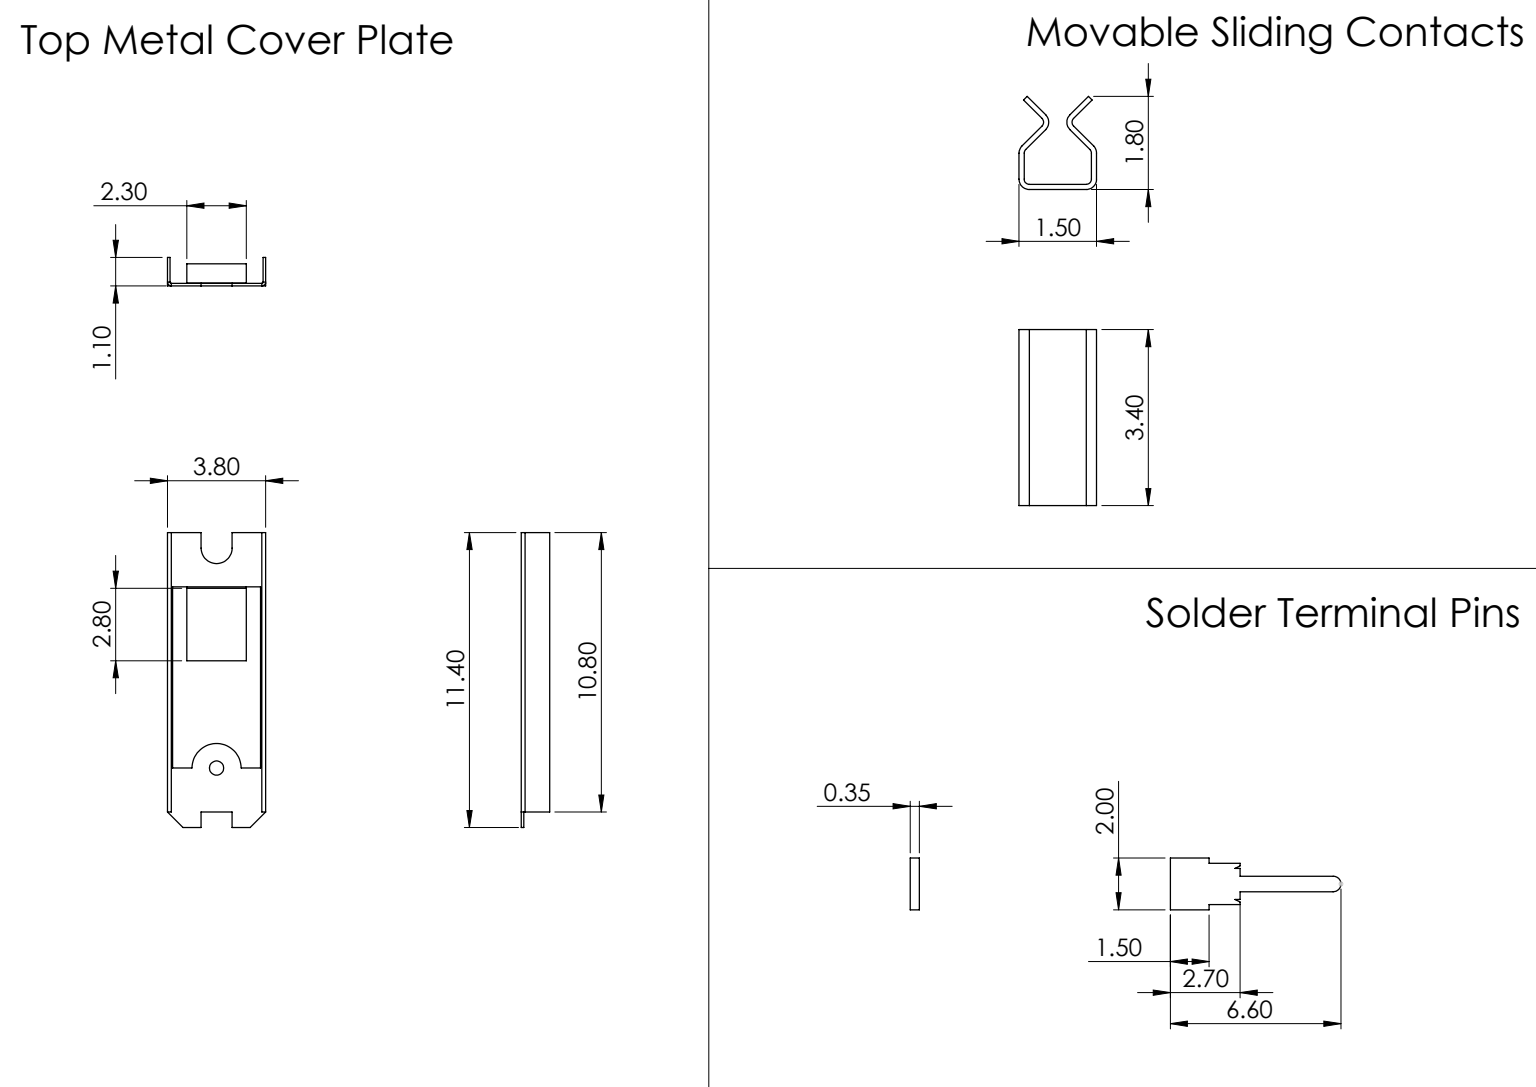
ISO-10303-21;
HEADER;
FILE_DESCRIPTION (('STEP AP214'),
    '1' );
FILE_NAME ('Movable Sliding Contacts.step',
    '2026-10-09T19:32:29',
    ( '' ),
    ( '' ),
    'SwSTEP 2.0',
    'SolidWorks 2026',
    '' );
FILE_SCHEMA (( 'AUTOMOTIVE_DESIGN' ));
ENDSEC;

DATA;
#11=DIRECTION ( 'NONE',  ( 1.306144734853129823E-16, -1.000000000000000000, -1.306144734853129823E-16 ) ) ;
#19=ORIENTED_EDGE ( 'NONE', *, *, #12813, .F. ) ;
#25=CARTESIAN_POINT ( 'NONE',  ( 0.3750000000000000000, 6.450000000000000178, 2.100000000000000089 ) ) ;
#54=CARTESIAN_POINT ( 'NONE',  ( 0.5500000000000000444, 6.450000000000000178, 3.399999999999999911 ) ) ;
#63=FACE_OUTER_BOUND ( 'NONE', #13945, .T. ) ;
#72=ORIENTED_EDGE ( 'NONE', *, *, #16562, .F. ) ;
#74=CARTESIAN_POINT ( 'NONE',  ( 0.5500000000000000444, 6.450000000000000178, 3.200000000000000178 ) ) ;
#100=DIRECTION ( 'NONE',  ( 1.306144734853129823E-16, -1.000000000000000000, -1.306144734853129823E-16 ) ) ;
#143=DIRECTION ( 'NONE',  ( 0.000000000000000000, -1.000000000000000000, -1.306144734853125878E-16 ) ) ;
#164=EDGE_LOOP ( 'NONE', ( #16318, #961, #5589, #9306 ) ) ;
#166=DIRECTION ( 'NONE',  ( 1.000000000000000000, 1.306144734853129823E-16, 0.000000000000000000 ) ) ;
#181=ORIENTED_EDGE ( 'NONE', *, *, #15801, .T. ) ;
#184=AXIS2_PLACEMENT_3D ( 'NONE', #11103, #16750, #840 ) ;
#200=FACE_OUTER_BOUND ( 'NONE', #10573, .T. ) ;
#206=DIRECTION ( 'NONE',  ( 1.142876642996489981E-16, -1.000000000000000000, -6.530723674265629391E-17 ) ) ;
#218=AXIS2_PLACEMENT_3D ( 'NONE', #8248, #6936, #4241 ) ;
#246=VECTOR ( 'NONE', #2226, 1000.000000000000000 ) ;
#258=ORIENTED_EDGE ( 'NONE', *, *, #12874, .T. ) ;
#268=VERTEX_POINT ( 'NONE', #877 ) ;
#269=LINE ( 'NONE', #7559, #15424 ) ;
#314=ORIENTED_EDGE ( 'NONE', *, *, #15602, .T. ) ;
#322=EDGE_CURVE ( 'NONE', #6911, #16493, #5032, .T. ) ;
#340=EDGE_CURVE ( 'NONE', #11433, #9105, #9389, .T. ) ;
#345=ORIENTED_EDGE ( 'NONE', *, *, #10185, .F. ) ;
#353=ORIENTED_EDGE ( 'NONE', *, *, #5292, .T. ) ;
#382=DIRECTION ( 'NONE',  ( 1.000000000000000000, 0.000000000000000000, 0.000000000000000000 ) ) ;
#433=CARTESIAN_POINT ( 'NONE',  ( 0.6207106781186549904, 3.050000000000000266, 2.628553390593269423 ) ) ;
#472=ADVANCED_FACE ( 'NONE', ( #11019 ), #9341, .T. ) ;
#507=CARTESIAN_POINT ( 'NONE',  ( -0.3750000000000000000, 3.050000000000000266, 2.100000000000000089 ) ) ;
#552=( GEOMETRIC_REPRESENTATION_CONTEXT ( 3 ) GLOBAL_UNCERTAINTY_ASSIGNED_CONTEXT ( ( #2517 ) ) GLOBAL_UNIT_ASSIGNED_CONTEXT ( ( #4504, #3040, #6174 ) ) REPRESENTATION_CONTEXT ( 'NONE', 'WORKASPACE' ) );
#554=DIRECTION ( 'NONE',  ( 1.306144734853129823E-16, -1.000000000000000000, -6.530723674265629391E-17 ) ) ;
#561=ADVANCED_FACE ( 'NONE', ( #4065 ), #6855, .F. ) ;
#606=CIRCLE ( 'NONE', #11850, 0.1999999999999999833 ) ;
#658=CARTESIAN_POINT ( 'NONE',  ( 0.6628679656440349399, 3.050000000000000266, 1.670710678118660031 ) ) ;
#668=DIRECTION ( 'NONE',  ( 0.7071067811865466846, 0.000000000000000000, -0.7071067811865483499 ) ) ;
#671=ORIENTED_EDGE ( 'NONE', *, *, #7463, .F. ) ;
#683=DIRECTION ( 'NONE',  ( 1.224646799147350002E-16, -1.000000000000000000, -6.123233995736769734E-17 ) ) ;
#686=ADVANCED_BREP_SHAPE_REPRESENTATION ( '', ( #7724, #17681 ), #552 ) ;
#696=PLANE ( 'NONE',  #836 ) ;
#706=ORIENTED_EDGE ( 'NONE', *, *, #14653, .F. ) ;
#724=ORIENTED_EDGE ( 'NONE', *, *, #11762, .T. ) ;
#741=EDGE_CURVE ( 'NONE', #9183, #17652, #3050, .T. ) ;
#758=EDGE_CURVE ( 'NONE', #16493, #14177, #16933, .T. ) ;
#771=VECTOR ( 'NONE', #10141, 1000.000000000000000 ) ;
#836=AXIS2_PLACEMENT_3D ( 'NONE', #6620, #6332, #10894 ) ;
#840=DIRECTION ( 'NONE',  ( 0.7071067811865594521, 0.000000000000000000, 0.7071067811865355823 ) ) ;
#845=ORIENTED_EDGE ( 'NONE', *, *, #5292, .F. ) ;
#877=CARTESIAN_POINT ( 'NONE',  ( 0.3042893218813449985, 3.050000000000000266, 2.170710678118660031 ) ) ;
#886=DIRECTION ( 'NONE',  ( -1.000000000000000000, 0.000000000000000000, 0.000000000000000000 ) ) ;
#931=FACE_OUTER_BOUND ( 'NONE', #3401, .T. ) ;
#949=CARTESIAN_POINT ( 'NONE',  ( -0.3042893218813459977, 6.450000000000000178, 2.029289321881350361 ) ) ;
#961=ORIENTED_EDGE ( 'NONE', *, *, #14653, .T. ) ;
#968=AXIS2_PLACEMENT_3D ( 'NONE', #5506, #11151, #6990 ) ;
#1018=ORIENTED_EDGE ( 'NONE', *, *, #16662, .T. ) ;
#1020=CARTESIAN_POINT ( 'NONE',  ( 0.6500000000000000222, 3.050000000000000266, 2.699264068711930253 ) ) ;
#1038=UNCERTAINTY_MEASURE_WITH_UNIT (LENGTH_MEASURE( 1.000000000000000082E-05 ), #15942, 'distance_accuracy_value', 'NONE');
#1043=CARTESIAN_POINT ( 'NONE',  ( -0.2335786437626909962, 6.450000000000000178, 2.241421356237310203 ) ) ;
#1070=DIRECTION ( 'NONE',  ( -1.224646799147351975E-16, 1.000000000000000000, 6.123233995736759873E-17 ) ) ;
#1079=LINE ( 'NONE', #17619, #15708 ) ;
#1081=DIRECTION ( 'NONE',  ( -1.224646799147350002E-16, 1.000000000000000000, 6.123233995736759873E-17 ) ) ;
#1100=VECTOR ( 'NONE', #13955, 1000.000000000000000 ) ;
#1118=CIRCLE ( 'NONE', #2598, 0.1000000000000000472 ) ;
#1147=ORIENTED_EDGE ( 'NONE', *, *, #10999, .T. ) ;
#1174=DIRECTION ( 'NONE',  ( -0.7071067811865475727, -4.040679121612663150E-17, -0.7071067811865475727 ) ) ;
#1182=DIRECTION ( 'NONE',  ( 1.000000000000000000, 0.000000000000000000, 0.000000000000000000 ) ) ;
#1198=CARTESIAN_POINT ( 'NONE',  ( -0.2335786437626909962, 6.450000000000000178, 2.241421356237310203 ) ) ;
#1199=ORIENTED_EDGE ( 'NONE', *, *, #2728, .T. ) ;
#1200=VECTOR ( 'NONE', #13384, 1000.000000000000000 ) ;
#1213=ADVANCED_FACE ( 'NONE', ( #2544 ), #12549, .T. ) ;
#1248=ORIENTED_EDGE ( 'NONE', *, *, #10846, .F. ) ;
#1251=DIRECTION ( 'NONE',  ( 0.7071067811865470176, -5.772398745161022854E-18, 0.7071067811865480168 ) ) ;
#1258=EDGE_CURVE ( 'NONE', #16824, #6139, #11523, .T. ) ;
#1283=ORIENTED_EDGE ( 'NONE', *, *, #4749, .F. ) ;
#1293=DIRECTION ( 'NONE',  ( -0.7071067811865475727, -4.617918996128746176E-17, -0.7071067811865475727 ) ) ;
#1324=ORIENTED_EDGE ( 'NONE', *, *, #3238, .F. ) ;
#1355=CARTESIAN_POINT ( 'NONE',  ( 0.5500000000000000444, 6.450000000000000178, 3.200000000000000178 ) ) ;
#1378=CARTESIAN_POINT ( 'NONE',  ( 0.6207106781186539912, 6.450000000000000178, 2.628553390593269423 ) ) ;
#1387=ORIENTED_EDGE ( 'NONE', *, *, #18174, .F. ) ;
#1400=AXIS2_PLACEMENT_3D ( 'NONE', #14762, #10784, #13285 ) ;
#1402=CIRCLE ( 'NONE', #3436, 0.2000000000000000389 ) ;
#1451=CARTESIAN_POINT ( 'NONE',  ( 0.6500000000000000222, 6.450000000000000178, 3.200000000000000178 ) ) ;
#1465=FACE_OUTER_BOUND ( 'NONE', #13748, .T. ) ;
#1483=VECTOR ( 'NONE', #3233, 1000.000000000000000 ) ;
#1498=ORIENTED_EDGE ( 'NONE', *, *, #12674, .T. ) ;
#1525=VECTOR ( 'NONE', #14731, 1000.000000000000000 ) ;
#1571=LINE ( 'NONE', #3365, #11024 ) ;
#1587=CARTESIAN_POINT ( 'NONE',  ( 0.5500000000000000444, 3.050000000000000266, 2.699264068711930253 ) ) ;
#1596=DIRECTION ( 'NONE',  ( -1.224646799147350002E-16, 1.000000000000000000, 6.123233995736759873E-17 ) ) ;
#1598=EDGE_CURVE ( 'NONE', #17652, #5170, #13115, .T. ) ;
#1676=DIRECTION ( 'NONE',  ( -1.224646799147350002E-16, 1.000000000000000000, 6.123233995736769734E-17 ) ) ;
#1749=CIRCLE ( 'NONE', #15946, 0.1000000000000000472 ) ;
#1753=DIRECTION ( 'NONE',  ( 1.306144734853129823E-16, -1.000000000000000000, -1.306144734853129823E-16 ) ) ;
#1766=ORIENTED_EDGE ( 'NONE', *, *, #11413, .T. ) ;
#1810=DIRECTION ( 'NONE',  ( 1.306144734853129823E-16, -1.000000000000000000, -1.306144734853129823E-16 ) ) ;
#1814=CARTESIAN_POINT ( 'NONE',  ( -0.5921572875253819923, 6.450000000000000178, 1.600000000000000089 ) ) ;
#1822=EDGE_CURVE ( 'NONE', #12759, #5909, #10605, .T. ) ;
#1842=DIRECTION ( 'NONE',  ( -0.7071067811865470176, 0.000000000000000000, -0.7071067811865480168 ) ) ;
#1881=EDGE_LOOP ( 'NONE', ( #8557, #7086, #17262, #671 ) ) ;
#1892=ORIENTED_EDGE ( 'NONE', *, *, #340, .T. ) ;
#1896=EDGE_CURVE ( 'NONE', #8650, #17860, #16398, .T. ) ;
#1922=CARTESIAN_POINT ( 'NONE',  ( -0.5921572875253809931, 3.050000000000000266, 1.600000000000000089 ) ) ;
#1976=DIRECTION ( 'NONE',  ( 0.7071067811865470176, 0.000000000000000000, -0.7071067811865480168 ) ) ;
#1982=AXIS2_PLACEMENT_3D ( 'NONE', #25, #8537, #5670 ) ;
#1984=AXIS2_PLACEMENT_3D ( 'NONE', #5604, #11249, #8735 ) ;
#1996=CARTESIAN_POINT ( 'NONE',  ( 0.5500000000000000444, 6.450000000000000178, 3.200000000000000178 ) ) ;
#2003=APPLICATION_CONTEXT ( 'automotive_design' ) ;
#2005=CARTESIAN_POINT ( 'NONE',  ( -0.6500000000000000222, 3.050000000000000266, 2.699264068711930253 ) ) ;
#2009=CIRCLE ( 'NONE', #5585, 0.09999999999999986677 ) ;
#2012=EDGE_CURVE ( 'NONE', #14546, #4205, #11057, .T. ) ;
#2075=FACE_OUTER_BOUND ( 'NONE', #17568, .T. ) ;
#2113=CARTESIAN_POINT ( 'NONE',  ( 0.2335786437626899970, 6.450000000000000178, 1.958578643762689753 ) ) ;
#2154=VECTOR ( 'NONE', #1976, 1000.000000000000000 ) ;
#2174=CYLINDRICAL_SURFACE ( 'NONE', #16153, 0.1999999999999999833 ) ;
#2226=DIRECTION ( 'NONE',  ( 0.7071067811865480168, 0.000000000000000000, 0.7071067811865470176 ) ) ;
#2229=EDGE_LOOP ( 'NONE', ( #6094, #10049, #6536, #13532 ) ) ;
#2239=ORIENTED_EDGE ( 'NONE', *, *, #15602, .F. ) ;
#2304=VERTEX_POINT ( 'NONE', #3612 ) ;
#2364=DIRECTION ( 'NONE',  ( -0.7071067811865480168, 0.000000000000000000, -0.7071067811865470176 ) ) ;
#2384=ORIENTED_EDGE ( 'NONE', *, *, #10846, .T. ) ;
#2386=CARTESIAN_POINT ( 'NONE',  ( 0.3750000000000000000, 6.450000000000000178, 2.100000000000000089 ) ) ;
#2392=DIRECTION ( 'NONE',  ( -0.7071067811865489050, 0.000000000000000000, 0.7071067811865461294 ) ) ;
#2397=CARTESIAN_POINT ( 'NONE',  ( 0.5500000000000000444, 3.050000000000000266, 2.699264068711930253 ) ) ;
#2432=ORIENTED_EDGE ( 'NONE', *, *, #18096, .F. ) ;
#2435=EDGE_LOOP ( 'NONE', ( #14296, #16546, #16833, #9896 ) ) ;
#2438=CARTESIAN_POINT ( 'NONE',  ( -0.6500000000000000222, 3.050000000000000266, 2.699264068711930253 ) ) ;
#2469=DIRECTION ( 'NONE',  ( -1.224646799147351975E-16, 1.000000000000000000, 6.123233995736750012E-17 ) ) ;
#2512=ADVANCED_FACE ( 'NONE', ( #16188 ), #14895, .T. ) ;
#2517=UNCERTAINTY_MEASURE_WITH_UNIT (LENGTH_MEASURE( 1.000000000000000082E-05 ), #4504, 'distance_accuracy_value', 'NONE');
#2521=CIRCLE ( 'NONE', #15240, 0.1999999999999999833 ) ;
#2544=FACE_OUTER_BOUND ( 'NONE', #16780, .T. ) ;
#2558=EDGE_LOOP ( 'NONE', ( #724, #14028, #6116, #7517 ) ) ;
#2583=DIRECTION ( 'NONE',  ( 1.224646799147350002E-16, -1.000000000000000000, -6.123233995736779594E-17 ) ) ;
#2598=AXIS2_PLACEMENT_3D ( 'NONE', #9789, #13865, #1182 ) ;
#2601=VECTOR ( 'NONE', #10358, 1000.000000000000000 ) ;
#2613=ORIENTED_EDGE ( 'NONE', *, *, #12876, .T. ) ;
#2645=AXIS2_PLACEMENT_3D ( 'NONE', #5227, #11989, #16247 ) ;
#2647=CARTESIAN_POINT ( 'NONE',  ( 0.6500000000000000222, 6.450000000000000178, 3.200000000000000178 ) ) ;
#2656=PLANE ( 'NONE',  #4452 ) ;
#2664=CARTESIAN_POINT ( 'NONE',  ( 0.2335786437626899970, 3.050000000000000266, 1.958578643762689753 ) ) ;
#2728=EDGE_CURVE ( 'NONE', #8832, #8965, #17864, .T. ) ;
#2741=DIRECTION ( 'NONE',  ( 1.224646799147350002E-16, -1.000000000000000000, -6.123233995736769734E-17 ) ) ;
#2742=VERTEX_POINT ( 'NONE', #17958 ) ;
#2772=CARTESIAN_POINT ( 'NONE',  ( 0.7500000000000000000, 6.450000000000000178, 2.699264068711930253 ) ) ;
#2841=EDGE_CURVE ( 'NONE', #12458, #7208, #6113, .T. ) ;
#2843=AXIS2_PLACEMENT_3D ( 'NONE', #12501, #13713, #13522 ) ;
#2844=CARTESIAN_POINT ( 'NONE',  ( 0.5500000000000000444, 6.450000000000000178, 3.299999999999999822 ) ) ;
#2861=VECTOR ( 'NONE', #3010, 1000.000000000000000 ) ;
#2873=VECTOR ( 'NONE', #1842, 1000.000000000000000 ) ;
#2895=CARTESIAN_POINT ( 'NONE',  ( 0.5500000000000000444, 6.450000000000000178, 2.699264068711930253 ) ) ;
#2930=VECTOR ( 'NONE', #15674, 1000.000000000000000 ) ;
#2941=ORIENTED_EDGE ( 'NONE', *, *, #13967, .T. ) ;
#2942=CIRCLE ( 'NONE', #12107, 0.2000000000000000389 ) ;
#2960=DIRECTION ( 'NONE',  ( -0.7071067811865475727, 0.000000000000000000, 0.7071067811865475727 ) ) ;
#2962=LINE ( 'NONE', #10082, #7056 ) ;
#2964=ORIENTED_EDGE ( 'NONE', *, *, #6783, .F. ) ;
#2991=CARTESIAN_POINT ( 'NONE',  ( 0.2335786437626899970, 3.050000000000000266, 2.241421356237310203 ) ) ;
#3010=DIRECTION ( 'NONE',  ( 1.306144734853129823E-16, -1.000000000000000000, 0.000000000000000000 ) ) ;
#3040=( NAMED_UNIT ( * ) PLANE_ANGLE_UNIT ( ) SI_UNIT ( $, .RADIAN. ) );
#3050=LINE ( 'NONE', #14338, #10224 ) ;
#3134=VECTOR ( 'NONE', #15451, 1000.000000000000000 ) ;
#3147=VECTOR ( 'NONE', #16065, 1000.000000000000000 ) ;
#3153=ADVANCED_FACE ( 'NONE', ( #15410 ), #14356, .T. ) ;
#3154=CARTESIAN_POINT ( 'NONE',  ( -0.2335786437626909962, 6.450000000000000178, 1.958578643762689753 ) ) ;
#3156=VECTOR ( 'NONE', #4485, 1000.000000000000000 ) ;
#3180=CARTESIAN_POINT ( 'NONE',  ( -0.6500000000000000222, 6.450000000000000178, 2.699264068711930253 ) ) ;
#3184=AXIS2_PLACEMENT_3D ( 'NONE', #9668, #2741, #4291 ) ;
#3186=AXIS2_PLACEMENT_3D ( 'NONE', #9689, #11361, #8490 ) ;
#3220=VERTEX_POINT ( 'NONE', #13993 ) ;
#3233=DIRECTION ( 'NONE',  ( -0.7071067811865480168, 0.000000000000000000, 0.7071067811865470176 ) ) ;
#3234=ORIENTED_EDGE ( 'NONE', *, *, #12205, .T. ) ;
#3238=EDGE_CURVE ( 'NONE', #16266, #4541, #14191, .T. ) ;
#3262=ADVANCED_FACE ( 'NONE', ( #200 ), #5844, .T. ) ;
#3336=ORIENTED_EDGE ( 'NONE', *, *, #14331, .F. ) ;
#3365=CARTESIAN_POINT ( 'NONE',  ( -0.7500000000000000000, 6.450000000000000178, 3.200000000000000178 ) ) ;
#3374=ORIENTED_EDGE ( 'NONE', *, *, #17726, .F. ) ;
#3386=ADVANCED_FACE ( 'NONE', ( #12278 ), #696, .T. ) ;
#3401=EDGE_LOOP ( 'NONE', ( #10796, #3614, #10052, #3336 ) ) ;
#3406=CARTESIAN_POINT ( 'NONE',  ( -0.6207106781186559896, 6.450000000000000178, 2.628553390593269423 ) ) ;
#3414=ORIENTED_EDGE ( 'NONE', *, *, #10999, .F. ) ;
#3421=ORIENTED_EDGE ( 'NONE', *, *, #14712, .F. ) ;
#3428=CARTESIAN_POINT ( 'NONE',  ( -0.5500000000000000444, 6.450000000000000178, 2.699264068711930253 ) ) ;
#3436=AXIS2_PLACEMENT_3D ( 'NONE', #6869, #7238, #16951 ) ;
#3448=VECTOR ( 'NONE', #4761, 1000.000000000000000 ) ;
#3450=AXIS2_PLACEMENT_3D ( 'NONE', #1355, #7011, #12660 ) ;
#3459=ADVANCED_FACE ( 'NONE', ( #10604 ), #7736, .F. ) ;
#3541=LINE ( 'NONE', #14852, #6231 ) ;
#3552=CARTESIAN_POINT ( 'NONE',  ( 0.2335786437626899970, 6.450000000000000178, 1.958578643762689753 ) ) ;
#3559=ORIENTED_EDGE ( 'NONE', *, *, #6783, .T. ) ;
#3565=ORIENTED_EDGE ( 'NONE', *, *, #9873, .F. ) ;
#3590=DIRECTION ( 'NONE',  ( -1.224646799147351975E-16, 1.000000000000000000, 6.123233995736750012E-17 ) ) ;
#3612=CARTESIAN_POINT ( 'NONE',  ( -0.5500000000000000444, 6.450000000000000178, 3.299999999999999822 ) ) ;
#3614=ORIENTED_EDGE ( 'NONE', *, *, #11569, .T. ) ;
#3658=VECTOR ( 'NONE', #7986, 1000.000000000000000 ) ;
#3673=EDGE_LOOP ( 'NONE', ( #10875, #11329, #8025, #12193 ) ) ;
#3691=CARTESIAN_POINT ( 'NONE',  ( 0.5500000000000000444, 3.050000000000000266, 3.299999999999999822 ) ) ;
#3702=ORIENTED_EDGE ( 'NONE', *, *, #9850, .F. ) ;
#3735=CARTESIAN_POINT ( 'NONE',  ( -0.5500000000000000444, 6.450000000000000178, 3.200000000000000178 ) ) ;
#3737=AXIS2_PLACEMENT_3D ( 'NONE', #16748, #1293, #4157 ) ;
#3781=ORIENTED_EDGE ( 'NONE', *, *, #9002, .F. ) ;
#3783=CYLINDRICAL_SURFACE ( 'NONE', #6371, 0.2000000000000000389 ) ;
#3787=VERTEX_POINT ( 'NONE', #4706 ) ;
#3809=VERTEX_POINT ( 'NONE', #16194 ) ;
#3880=AXIS2_PLACEMENT_3D ( 'NONE', #4906, #17861, #13537 ) ;
#3907=ORIENTED_EDGE ( 'NONE', *, *, #1258, .F. ) ;
#3920=EDGE_CURVE ( 'NONE', #3809, #14294, #17386, .T. ) ;
#3949=CARTESIAN_POINT ( 'NONE',  ( 0.3042893218813439438, 6.450000000000000178, 2.170710678118660031 ) ) ;
#3984=ADVANCED_FACE ( 'NONE', ( #11094 ), #3783, .T. ) ;
#4034=VECTOR ( 'NONE', #4386, 1000.000000000000000 ) ;
#4051=VECTOR ( 'NONE', #1810, 1000.000000000000000 ) ;
#4065=FACE_OUTER_BOUND ( 'NONE', #2435, .T. ) ;
#4113=AXIS2_PLACEMENT_3D ( 'NONE', #507, #5981, #11622 ) ;
#4125=CARTESIAN_POINT ( 'NONE',  ( 0.5500000000000000444, 3.050000000000000266, 3.399999999999999911 ) ) ;
#4141=FACE_OUTER_BOUND ( 'NONE', #11507, .T. ) ;
#4146=DIRECTION ( 'NONE',  ( 1.000000000000000000, 0.000000000000000000, 0.000000000000000000 ) ) ;
#4153=CARTESIAN_POINT ( 'NONE',  ( -0.2335786437626909962, 3.050000000000000266, 1.958578643762689753 ) ) ;
#4157=DIRECTION ( 'NONE',  ( -0.7071067811865475727, 0.000000000000000000, 0.7071067811865475727 ) ) ;
#4169=CARTESIAN_POINT ( 'NONE',  ( -0.5500000000000000444, 3.050000000000000266, 3.299999999999999822 ) ) ;
#4205=VERTEX_POINT ( 'NONE', #8540 ) ;
#4213=DIRECTION ( 'NONE',  ( -0.7071067811865475727, 0.000000000000000000, 0.7071067811865475727 ) ) ;
#4216=EDGE_CURVE ( 'NONE', #11075, #16312, #8486, .T. ) ;
#4220=CYLINDRICAL_SURFACE ( 'NONE', #3450, 0.09999999999999982514 ) ;
#4241=DIRECTION ( 'NONE',  ( 0.000000000000000000, 0.000000000000000000, 1.000000000000000000 ) ) ;
#4291=DIRECTION ( 'NONE',  ( 0.000000000000000000, 0.000000000000000000, 1.000000000000000000 ) ) ;
#4314=DIRECTION ( 'NONE',  ( 1.000000000000000000, 0.000000000000000000, 0.000000000000000000 ) ) ;
#4323=DIRECTION ( 'NONE',  ( -1.306144734853129823E-16, 1.000000000000000000, 0.000000000000000000 ) ) ;
#4325=AXIS2_PLACEMENT_3D ( 'NONE', #3428, #6761, #9080 ) ;
#4360=ADVANCED_FACE ( 'NONE', ( #8709 ), #14354, .F. ) ;
#4386=DIRECTION ( 'NONE',  ( 0.000000000000000000, 0.000000000000000000, 1.000000000000000000 ) ) ;
#4446=( NAMED_UNIT ( * ) SI_UNIT ( $, .STERADIAN. ) SOLID_ANGLE_UNIT ( ) );
#4452=AXIS2_PLACEMENT_3D ( 'NONE', #1451, #6823, #18085 ) ;
#4466=EDGE_LOOP ( 'NONE', ( #15778, #10124, #4686, #12944 ) ) ;
#4485=DIRECTION ( 'NONE',  ( 0.000000000000000000, 0.000000000000000000, 1.000000000000000000 ) ) ;
#4487=CARTESIAN_POINT ( 'NONE',  ( 0.6628679656440349399, 6.450000000000000178, 1.670710678118660031 ) ) ;
#4504=( LENGTH_UNIT ( ) NAMED_UNIT ( * ) SI_UNIT ( .MILLI., .METRE. ) );
#4541=VERTEX_POINT ( 'NONE', #3691 ) ;
#4614=SHAPE_REPRESENTATION ( 'Movable Sliding Contacts', ( #17681 ), #552 ) ;
#4632=ORIENTED_EDGE ( 'NONE', *, *, #4865, .T. ) ;
#4645=ORIENTED_EDGE ( 'NONE', *, *, #2841, .T. ) ;
#4683=LINE ( 'NONE', #17177, #9778 ) ;
#4686=ORIENTED_EDGE ( 'NONE', *, *, #16963, .F. ) ;
#4687=LINE ( 'NONE', #17181, #5937 ) ;
#4689=CARTESIAN_POINT ( 'NONE',  ( -0.7500000000000000000, 6.450000000000000178, 3.200000000000000178 ) ) ;
#4706=CARTESIAN_POINT ( 'NONE',  ( -0.7500000000000000000, 3.050000000000000266, 3.200000000000000178 ) ) ;
#4720=CIRCLE ( 'NONE', #13618, 0.09999999999999990841 ) ;
#4721=DIRECTION ( 'NONE',  ( 1.306144734853129823E-16, -1.000000000000000000, -1.306144734853129823E-16 ) ) ;
#4749=EDGE_CURVE ( 'NONE', #17050, #8650, #2521, .T. ) ;
#4761=DIRECTION ( 'NONE',  ( 0.000000000000000000, 0.000000000000000000, -1.000000000000000000 ) ) ;
#4766=DIRECTION ( 'NONE',  ( -1.224646799147350002E-16, 1.000000000000000000, 6.123233995736769734E-17 ) ) ;
#4774=CARTESIAN_POINT ( 'NONE',  ( -0.6628679656440360501, 3.050000000000000266, 1.670710678118650261 ) ) ;
#4864=ORIENTED_EDGE ( 'NONE', *, *, #8470, .F. ) ;
#4865=EDGE_CURVE ( 'NONE', #6673, #3787, #1571, .T. ) ;
#4895=LINE ( 'NONE', #16209, #246 ) ;
#4897=LINE ( 'NONE', #11582, #11520 ) ;
#4905=ORIENTED_EDGE ( 'NONE', *, *, #14101, .T. ) ;
#4906=CARTESIAN_POINT ( 'NONE',  ( 0.5500000000000000444, 3.050000000000000266, 3.200000000000000178 ) ) ;
#4909=CARTESIAN_POINT ( 'NONE',  ( 0.7500000000000000000, 6.450000000000000178, 2.699264068711930253 ) ) ;
#4924=EDGE_CURVE ( 'NONE', #6699, #16493, #11985, .T. ) ;
#4939=CARTESIAN_POINT ( 'NONE',  ( -0.6628679656440360501, 3.050000000000000266, 1.670710678118650261 ) ) ;
#4953=LINE ( 'NONE', #10503, #7999 ) ;
#4989=CARTESIAN_POINT ( 'NONE',  ( 0.7500000000000000000, 6.450000000000000178, 3.200000000000000178 ) ) ;
#5032=LINE ( 'NONE', #6409, #16724 ) ;
#5069=EDGE_LOOP ( 'NONE', ( #6880, #1766, #3565, #14702 ) ) ;
#5072=LINE ( 'NONE', #14992, #7068 ) ;
#5096=ORIENTED_EDGE ( 'NONE', *, *, #2841, .F. ) ;
#5102=ORIENTED_EDGE ( 'NONE', *, *, #13168, .T. ) ;
#5150=VERTEX_POINT ( 'NONE', #16702 ) ;
#5170=VERTEX_POINT ( 'NONE', #10045 ) ;
#5227=CARTESIAN_POINT ( 'NONE',  ( -0.5500000000000000444, 6.450000000000000178, 3.200000000000000178 ) ) ;
#5244=DIRECTION ( 'NONE',  ( 1.000000000000000000, 0.000000000000000000, 0.000000000000000000 ) ) ;
#5263=AXIS2_PLACEMENT_3D ( 'NONE', #14963, #1070, #7824 ) ;
#5276=VECTOR ( 'NONE', #16361, 1000.000000000000000 ) ;
#5280=VECTOR ( 'NONE', #7789, 1000.000000000000000 ) ;
#5292=EDGE_CURVE ( 'NONE', #14118, #3787, #11760, .T. ) ;
#5404=DIRECTION ( 'NONE',  ( 1.306144734853129823E-16, -1.000000000000000000, -1.306144734853129823E-16 ) ) ;
#5454=CARTESIAN_POINT ( 'NONE',  ( -0.3750000000000000000, 6.450000000000000178, 2.100000000000000089 ) ) ;
#5506=CARTESIAN_POINT ( 'NONE',  ( 0.6207106781186539912, 6.450000000000000178, 2.628553390593269423 ) ) ;
#5523=LINE ( 'NONE', #10062, #3156 ) ;
#5585=AXIS2_PLACEMENT_3D ( 'NONE', #11956, #14552, #14633 ) ;
#5589=ORIENTED_EDGE ( 'NONE', *, *, #17058, .F. ) ;
#5604=CARTESIAN_POINT ( 'NONE',  ( -0.5500000000000000444, 3.050000000000000266, 3.200000000000000178 ) ) ;
#5670=DIRECTION ( 'NONE',  ( -0.7071067811865489050, 0.000000000000000000, 0.7071067811865461294 ) ) ;
#5675=DIRECTION ( 'NONE',  ( 1.224646799147351975E-16, -1.000000000000000000, -6.123233995736789455E-17 ) ) ;
#5697=CARTESIAN_POINT ( 'NONE',  ( 0.6500000000000000222, 6.450000000000000178, 2.699264068711930253 ) ) ;
#5746=EDGE_CURVE ( 'NONE', #9328, #14177, #12889, .T. ) ;
#5760=DIRECTION ( 'NONE',  ( 0.7071067811865466846, 0.000000000000000000, -0.7071067811865483499 ) ) ;
#5774=EDGE_CURVE ( 'NONE', #7292, #12458, #4895, .T. ) ;
#5786=DIRECTION ( 'NONE',  ( -1.000000000000000000, 0.000000000000000000, 0.000000000000000000 ) ) ;
#5831=DIRECTION ( 'NONE',  ( 1.224646799147351975E-16, -1.000000000000000000, -6.123233995736789455E-17 ) ) ;
#5834=CARTESIAN_POINT ( 'NONE',  ( 0.5500000000000000444, 6.450000000000000178, 3.399999999999999911 ) ) ;
#5835=COLOUR_RGB ( '', 0.40784314, 0.44705882, 0.49803922) ;
#5839=PRESENTATION_STYLE_ASSIGNMENT (( #13060 ) ) ;
#5844=PLANE ( 'NONE',  #16799 ) ;
#5845=CARTESIAN_POINT ( 'NONE',  ( 0.7500000000000000000, 6.450000000000000178, 2.699264068711930253 ) ) ;
#5870=VECTOR ( 'NONE', #5404, 1000.000000000000000 ) ;
#5909=VERTEX_POINT ( 'NONE', #16034 ) ;
#5933=DIRECTION ( 'NONE',  ( 1.632680918566409751E-16, -1.000000000000000000, -1.306144734853129823E-16 ) ) ;
#5935=DIRECTION ( 'NONE',  ( 0.000000000000000000, -1.000000000000000000, -1.306144734853123906E-16 ) ) ;
#5937=VECTOR ( 'NONE', #10340, 1000.000000000000000 ) ;
#5959=CARTESIAN_POINT ( 'NONE',  ( -0.6628679656440369383, 6.450000000000000178, 1.670710678118660031 ) ) ;
#5967=DIRECTION ( 'NONE',  ( 1.000000000000000000, 0.000000000000000000, 0.000000000000000000 ) ) ;
#5981=DIRECTION ( 'NONE',  ( -1.224646799147350002E-16, 1.000000000000000000, 6.123233995736759873E-17 ) ) ;
#6028=ORIENTED_EDGE ( 'NONE', *, *, #741, .F. ) ;
#6052=CARTESIAN_POINT ( 'NONE',  ( -0.5500000000000000444, 6.450000000000000178, 3.299999999999999822 ) ) ;
#6064=CARTESIAN_POINT ( 'NONE',  ( -0.7500000000000000000, 3.050000000000000266, 3.200000000000000178 ) ) ;
#6094=ORIENTED_EDGE ( 'NONE', *, *, #12109, .T. ) ;
#6100=FACE_OUTER_BOUND ( 'NONE', #10115, .T. ) ;
#6113=CIRCLE ( 'NONE', #16520, 0.2000000000000000389 ) ;
#6116=ORIENTED_EDGE ( 'NONE', *, *, #12874, .F. ) ;
#6123=ORIENTED_EDGE ( 'NONE', *, *, #8168, .F. ) ;
#6139=VERTEX_POINT ( 'NONE', #11562 ) ;
#6140=LINE ( 'NONE', #17425, #4051 ) ;
#6168=DIRECTION ( 'NONE',  ( 1.306144734853129823E-16, -1.000000000000000000, 0.000000000000000000 ) ) ;
#6174=( NAMED_UNIT ( * ) SI_UNIT ( $, .STERADIAN. ) SOLID_ANGLE_UNIT ( ) );
#6184=LINE ( 'NONE', #11840, #2873 ) ;
#6206=DIRECTION ( 'NONE',  ( 0.7071067811865470176, 9.235837992257496050E-17, -0.7071067811865480168 ) ) ;
#6214=VERTEX_POINT ( 'NONE', #14064 ) ;
#6231=VECTOR ( 'NONE', #10773, 1000.000000000000000 ) ;
#6239=CARTESIAN_POINT ( 'NONE',  ( -0.5500000000000000444, 6.450000000000000178, 2.699264068711930253 ) ) ;
#6255=LINE ( 'NONE', #11725, #15993 ) ;
#6270=CARTESIAN_POINT ( 'NONE',  ( -0.6500000000000000222, 6.450000000000000178, 2.699264068711930253 ) ) ;
#6289=ORIENTED_EDGE ( 'NONE', *, *, #758, .T. ) ;
#6324=DIRECTION ( 'NONE',  ( -1.306144734853129823E-16, 1.000000000000000000, 0.000000000000000000 ) ) ;
#6332=DIRECTION ( 'NONE',  ( 0.000000000000000000, 1.306144734853129823E-16, -1.000000000000000000 ) ) ;
#6371=AXIS2_PLACEMENT_3D ( 'NONE', #5454, #2583, #12307 ) ;
#6383=LINE ( 'NONE', #658, #5280 ) ;
#6396=ORIENTED_EDGE ( 'NONE', *, *, #15381, .F. ) ;
#6409=CARTESIAN_POINT ( 'NONE',  ( -0.5921572875253819923, 6.450000000000000178, 1.600000000000000089 ) ) ;
#6420=CYLINDRICAL_SURFACE ( 'NONE', #2645, 0.2000000000000000944 ) ;
#6476=EDGE_CURVE ( 'NONE', #8985, #11075, #2962, .T. ) ;
#6493=EDGE_LOOP ( 'NONE', ( #10469, #2613, #345, #4864 ) ) ;
#6496=SHAPE_DEFINITION_REPRESENTATION ( #10670, #4614 ) ;
#6502=AXIS2_PLACEMENT_3D ( 'NONE', #12671, #13876, #11456 ) ;
#6523=ADVANCED_FACE ( 'NONE', ( #15554 ), #16925, .T. ) ;
#6528=AXIS2_PLACEMENT_3D ( 'NONE', #16923, #11093, #2960 ) ;
#6536=ORIENTED_EDGE ( 'NONE', *, *, #758, .F. ) ;
#6553=CARTESIAN_POINT ( 'NONE',  ( -0.2335786437626909962, 6.450000000000000178, 1.958578643762689753 ) ) ;
#6570=PLANE ( 'NONE',  #18247 ) ;
#6620=CARTESIAN_POINT ( 'NONE',  ( -0.5500000000000000444, 6.450000000000000178, 3.299999999999999822 ) ) ;
#6628=CARTESIAN_POINT ( 'NONE',  ( -0.6207106781186549904, 3.050000000000000266, 2.628553390593269423 ) ) ;
#6654=CARTESIAN_POINT ( 'NONE',  ( 0.2335786437626899970, 6.450000000000000178, 1.958578643762689753 ) ) ;
#6673=VERTEX_POINT ( 'NONE', #4689 ) ;
#6699=VERTEX_POINT ( 'NONE', #4774 ) ;
#6739=ORIENTED_EDGE ( 'NONE', *, *, #8168, .T. ) ;
#6761=DIRECTION ( 'NONE',  ( 1.224646799147350002E-16, -1.000000000000000000, -6.123233995736769734E-17 ) ) ;
#6783=EDGE_CURVE ( 'NONE', #16266, #10138, #11739, .T. ) ;
#6808=FACE_OUTER_BOUND ( 'NONE', #16571, .T. ) ;
#6812=ORIENTED_EDGE ( 'NONE', *, *, #14840, .T. ) ;
#6817=VECTOR ( 'NONE', #6168, 1000.000000000000000 ) ;
#6823=DIRECTION ( 'NONE',  ( -1.000000000000000000, -1.306144734853129823E-16, 0.000000000000000000 ) ) ;
#6855=CYLINDRICAL_SURFACE ( 'NONE', #184, 0.09999999999999997780 ) ;
#6869=CARTESIAN_POINT ( 'NONE',  ( 0.3750000000000000000, 6.450000000000000178, 2.100000000000000089 ) ) ;
#6880=ORIENTED_EDGE ( 'NONE', *, *, #14712, .T. ) ;
#6891=VERTEX_POINT ( 'NONE', #6628 ) ;
#6903=AXIS2_PLACEMENT_3D ( 'NONE', #9114, #4766, #17528 ) ;
#6911=VERTEX_POINT ( 'NONE', #8580 ) ;
#6936=DIRECTION ( 'NONE',  ( -1.224646799147350002E-16, 1.000000000000000000, 6.123233995736759873E-17 ) ) ;
#6951=LINE ( 'NONE', #4169, #10366 ) ;
#6990=DIRECTION ( 'NONE',  ( -1.306144734853125878E-16, 1.000000000000000000, 0.000000000000000000 ) ) ;
#7011=DIRECTION ( 'NONE',  ( -1.224646799147350002E-16, 1.000000000000000000, 6.123233995736769734E-17 ) ) ;
#7027=AXIS2_PLACEMENT_3D ( 'NONE', #54, #18073, #13936 ) ;
#7056=VECTOR ( 'NONE', #17182, 1000.000000000000000 ) ;
#7068=VECTOR ( 'NONE', #12210, 1000.000000000000000 ) ;
#7071=DIRECTION ( 'NONE',  ( 1.306144734853129823E-16, -1.000000000000000000, -1.306144734853129823E-16 ) ) ;
#7086=ORIENTED_EDGE ( 'NONE', *, *, #3920, .T. ) ;
#7091=ORIENTED_EDGE ( 'NONE', *, *, #14840, .F. ) ;
#7099=ORIENTED_EDGE ( 'NONE', *, *, #3920, .F. ) ;
#7123=EDGE_CURVE ( 'NONE', #4205, #14294, #5523, .T. ) ;
#7199=CARTESIAN_POINT ( 'NONE',  ( 0.3042893218813449985, 3.050000000000000266, 2.170710678118660031 ) ) ;
#7208=VERTEX_POINT ( 'NONE', #11267 ) ;
#7231=LINE ( 'NONE', #5834, #2930 ) ;
#7238=DIRECTION ( 'NONE',  ( 1.224646799147350002E-16, -1.000000000000000000, -6.123233995736779594E-17 ) ) ;
#7240=DIRECTION ( 'NONE',  ( 0.7071067811865594521, 0.000000000000000000, 0.7071067811865355823 ) ) ;
#7285=ORIENTED_EDGE ( 'NONE', *, *, #2012, .F. ) ;
#7292=VERTEX_POINT ( 'NONE', #9075 ) ;
#7294=DIRECTION ( 'NONE',  ( 0.7071067811865470176, 0.000000000000000000, 0.7071067811865480168 ) ) ;
#7330=DIRECTION ( 'NONE',  ( 0.000000000000000000, 0.000000000000000000, 1.000000000000000000 ) ) ;
#7390=CARTESIAN_POINT ( 'NONE',  ( -0.5500000000000000444, 3.050000000000000266, 2.699264068711930253 ) ) ;
#7400=CARTESIAN_POINT ( 'NONE',  ( -0.3042893218813459977, 6.450000000000000178, 2.029289321881350361 ) ) ;
#7407=CARTESIAN_POINT ( 'NONE',  ( 0.6628679656440349399, 6.450000000000000178, 1.670710678118660031 ) ) ;
#7443=ORIENTED_EDGE ( 'NONE', *, *, #1822, .T. ) ;
#7463=EDGE_CURVE ( 'NONE', #7208, #4205, #16127, .T. ) ;
#7468=LINE ( 'NONE', #6064, #3448 ) ;
#7469=DIRECTION ( 'NONE',  ( -0.7071067811865480168, 0.000000000000000000, 0.7071067811865470176 ) ) ;
#7473=DIRECTION ( 'NONE',  ( -1.224646799147351975E-16, 1.000000000000000000, 6.123233995736759873E-17 ) ) ;
#7517=ORIENTED_EDGE ( 'NONE', *, *, #10613, .F. ) ;
#7532=FACE_OUTER_BOUND ( 'NONE', #2229, .T. ) ;
#7559=CARTESIAN_POINT ( 'NONE',  ( 0.5921572875253799939, 6.450000000000000178, 1.600000000000000089 ) ) ;
#7606=VECTOR ( 'NONE', #1753, 1000.000000000000000 ) ;
#7614=ORIENTED_EDGE ( 'NONE', *, *, #8952, .F. ) ;
#7620=ORIENTED_EDGE ( 'NONE', *, *, #12760, .T. ) ;
#7627=LINE ( 'NONE', #10398, #10306 ) ;
#7649=LINE ( 'NONE', #16000, #6817 ) ;
#7674=ORIENTED_EDGE ( 'NONE', *, *, #322, .T. ) ;
#7686=ADVANCED_FACE ( 'NONE', ( #13989 ), #12602, .T. ) ;
#7701=LINE ( 'NONE', #949, #17456 ) ;
#7717=ORIENTED_EDGE ( 'NONE', *, *, #15478, .F. ) ;
#7718=CIRCLE ( 'NONE', #3880, 0.1999999999999999833 ) ;
#7724=MANIFOLD_SOLID_BREP ( 'Stock-MAS-687-1', #10526 ) ;
#7736=CYLINDRICAL_SURFACE ( 'NONE', #13523, 0.09999999999999986677 ) ;
#7749=CARTESIAN_POINT ( 'NONE',  ( -0.3750000000000000000, 6.450000000000000178, 2.100000000000000089 ) ) ;
#7756=CARTESIAN_POINT ( 'NONE',  ( -0.2335786437626909962, 3.050000000000000266, 2.241421356237310203 ) ) ;
#7789=DIRECTION ( 'NONE',  ( -0.7071067811865480168, 0.000000000000000000, 0.7071067811865470176 ) ) ;
#7792=LINE ( 'NONE', #9073, #1525 ) ;
#7806=DIRECTION ( 'NONE',  ( 0.7071067811865489050, 0.000000000000000000, 0.7071067811865460184 ) ) ;
#7820=LINE ( 'NONE', #3552, #8839 ) ;
#7824=DIRECTION ( 'NONE',  ( -0.7071067811865500152, 0.000000000000000000, -0.7071067811865451302 ) ) ;
#7847=CARTESIAN_POINT ( 'NONE',  ( -0.6207106781186559896, 6.450000000000000178, 2.628553390593269423 ) ) ;
#7916=CIRCLE ( 'NONE', #1400, 0.09999999999999990841 ) ;
#7939=VERTEX_POINT ( 'NONE', #1020 ) ;
#7953=ADVANCED_FACE ( 'NONE', ( #931 ), #6570, .T. ) ;
#7960=AXIS2_PLACEMENT_3D ( 'NONE', #11834, #17266, #8953 ) ;
#7964=CARTESIAN_POINT ( 'NONE',  ( -0.5500000000000000444, 6.450000000000000178, 2.699264068711930253 ) ) ;
#7986=DIRECTION ( 'NONE',  ( 0.7071067811865480168, 0.000000000000000000, -0.7071067811865470176 ) ) ;
#7989=ORIENTED_EDGE ( 'NONE', *, *, #18096, .T. ) ;
#7991=ORIENTED_EDGE ( 'NONE', *, *, #11332, .T. ) ;
#7994=DIRECTION ( 'NONE',  ( 1.306144734853129823E-16, -1.000000000000000000, 0.000000000000000000 ) ) ;
#7999=VECTOR ( 'NONE', #9116, 1000.000000000000000 ) ;
#8021=PRODUCT ( 'Movable Sliding Contacts', 'Movable Sliding Contacts', '', ( #13442 ) ) ;
#8025=ORIENTED_EDGE ( 'NONE', *, *, #13168, .F. ) ;
#8046=DIRECTION ( 'NONE',  ( 0.7071067811865489050, 0.000000000000000000, -0.7071067811865461294 ) ) ;
#8077=ORIENTED_EDGE ( 'NONE', *, *, #12674, .F. ) ;
#8129=LINE ( 'NONE', #3949, #3134 ) ;
#8166=CARTESIAN_POINT ( 'NONE',  ( -0.5500000000000000444, 6.450000000000000178, 3.399999999999999911 ) ) ;
#8168=EDGE_CURVE ( 'NONE', #12909, #17652, #12115, .T. ) ;
#8194=FACE_OUTER_BOUND ( 'NONE', #6493, .T. ) ;
#8204=MECHANICAL_DESIGN_GEOMETRIC_PRESENTATION_REPRESENTATION('',(#15623),#15315);
#8211=ORIENTED_EDGE ( 'NONE', *, *, #15478, .T. ) ;
#8224=AXIS2_PLACEMENT_3D ( 'NONE', #17811, #16354, #2392 ) ;
#8248=CARTESIAN_POINT ( 'NONE',  ( 0.5500000000000000444, 3.050000000000000266, 3.200000000000000178 ) ) ;
#8263=ORIENTED_EDGE ( 'NONE', *, *, #13790, .T. ) ;
#8287=EDGE_LOOP ( 'NONE', ( #12217, #8263, #9803, #8564 ) ) ;
#8399=ORIENTED_EDGE ( 'NONE', *, *, #10613, .T. ) ;
#8470=EDGE_CURVE ( 'NONE', #16824, #12466, #7231, .T. ) ;
#8484=ORIENTED_EDGE ( 'NONE', *, *, #17947, .T. ) ;
#8486=CIRCLE ( 'NONE', #13247, 0.09999999999999997780 ) ;
#8490=DIRECTION ( 'NONE',  ( 0.7071067811865489050, 0.000000000000000000, -0.7071067811865461294 ) ) ;
#8492=LINE ( 'NONE', #7199, #1100 ) ;
#8537=DIRECTION ( 'NONE',  ( 1.224646799147350002E-16, -1.000000000000000000, -6.123233995736779594E-17 ) ) ;
#8540=CARTESIAN_POINT ( 'NONE',  ( 0.7500000000000000000, 3.050000000000000266, 2.699264068711930253 ) ) ;
#8557=ORIENTED_EDGE ( 'NONE', *, *, #8952, .T. ) ;
#8564=ORIENTED_EDGE ( 'NONE', *, *, #17947, .F. ) ;
#8579=AXIS2_PLACEMENT_3D ( 'NONE', #7964, #3590, #17924 ) ;
#8580=CARTESIAN_POINT ( 'NONE',  ( -0.5921572875253819923, 6.450000000000000178, 1.600000000000000089 ) ) ;
#8599=EDGE_LOOP ( 'NONE', ( #1018, #4632, #845, #11955 ) ) ;
#8650=VERTEX_POINT ( 'NONE', #11758 ) ;
#8668=ORIENTED_EDGE ( 'NONE', *, *, #5774, .F. ) ;
#8706=LINE ( 'NONE', #8971, #11508 ) ;
#8709=FACE_OUTER_BOUND ( 'NONE', #5069, .T. ) ;
#8729=ORIENTED_EDGE ( 'NONE', *, *, #2012, .T. ) ;
#8735=DIRECTION ( 'NONE',  ( 0.000000000000000000, 0.000000000000000000, 1.000000000000000000 ) ) ;
#8775=CARTESIAN_POINT ( 'NONE',  ( 0.7500000000000000000, 3.050000000000000266, 3.200000000000000178 ) ) ;
#8777=AXIS2_PLACEMENT_3D ( 'NONE', #16717, #1081, #13483 ) ;
#8832=VERTEX_POINT ( 'NONE', #1198 ) ;
#8839=VECTOR ( 'NONE', #17797, 1000.000000000000000 ) ;
#8868=ORIENTED_EDGE ( 'NONE', *, *, #11413, .F. ) ;
#8884=VERTEX_POINT ( 'NONE', #6654 ) ;
#8887=SURFACE_SIDE_STYLE ('',( #17288 ) ) ;
#8916=LINE ( 'NONE', #5845, #16818 ) ;
#8952=EDGE_CURVE ( 'NONE', #7208, #3809, #8916, .T. ) ;
#8953=DIRECTION ( 'NONE',  ( 0.000000000000000000, 6.123233995736769734E-17, -1.000000000000000000 ) ) ;
#8965=VERTEX_POINT ( 'NONE', #7756 ) ;
#8971=CARTESIAN_POINT ( 'NONE',  ( 0.5921572875253799939, 6.450000000000000178, 1.600000000000000089 ) ) ;
#8975=CARTESIAN_POINT ( 'NONE',  ( 0.5500000000000000444, 6.450000000000000178, 2.699264068711930253 ) ) ;
#8981=ORIENTED_EDGE ( 'NONE', *, *, #10322, .F. ) ;
#8985=VERTEX_POINT ( 'NONE', #14457 ) ;
#8998=ORIENTED_EDGE ( 'NONE', *, *, #11534, .F. ) ;
#9002=EDGE_CURVE ( 'NONE', #9183, #2304, #1749, .T. ) ;
#9070=CIRCLE ( 'NONE', #3184, 0.2000000000000000944 ) ;
#9073=CARTESIAN_POINT ( 'NONE',  ( 0.6628679656440349399, 6.450000000000000178, 1.670710678118660031 ) ) ;
#9075=CARTESIAN_POINT ( 'NONE',  ( 0.3042893218813439438, 6.450000000000000178, 2.170710678118660031 ) ) ;
#9080=DIRECTION ( 'NONE',  ( -1.000000000000000000, 0.000000000000000000, 0.000000000000000000 ) ) ;
#9083=ORIENTED_EDGE ( 'NONE', *, *, #12109, .F. ) ;
#9102=CARTESIAN_POINT ( 'NONE',  ( -0.7500000000000000000, 6.450000000000000178, 3.200000000000000178 ) ) ;
#9105=VERTEX_POINT ( 'NONE', #2991 ) ;
#9114=CARTESIAN_POINT ( 'NONE',  ( -0.5500000000000000444, 3.050000000000000266, 3.200000000000000178 ) ) ;
#9116=DIRECTION ( 'NONE',  ( 1.306144734853129823E-16, -1.000000000000000000, -1.306144734853129823E-16 ) ) ;
#9142=DIRECTION ( 'NONE',  ( 1.224510688924809779E-16, -1.000000000000000000, -6.530723674265629391E-17 ) ) ;
#9165=VERTEX_POINT ( 'NONE', #14357 ) ;
#9169=ORIENTED_EDGE ( 'NONE', *, *, #5774, .T. ) ;
#9183=VERTEX_POINT ( 'NONE', #13868 ) ;
#9196=DIRECTION ( 'NONE',  ( 1.306144734853129823E-16, -1.000000000000000000, -1.306144734853129823E-16 ) ) ;
#9239=VERTEX_POINT ( 'NONE', #7847 ) ;
#9306=ORIENTED_EDGE ( 'NONE', *, *, #1822, .F. ) ;
#9328=VERTEX_POINT ( 'NONE', #6553 ) ;
#9334=VECTOR ( 'NONE', #15826, 1000.000000000000000 ) ;
#9341=PLANE ( 'NONE',  #2843 ) ;
#9350=CARTESIAN_POINT ( 'NONE',  ( -0.6914213562373099364, 3.050000000000000266, 2.557842712474620139 ) ) ;
#9351=VERTEX_POINT ( 'NONE', #16558 ) ;
#9372=ORIENTED_EDGE ( 'NONE', *, *, #12249, .T. ) ;
#9374=AXIS2_PLACEMENT_3D ( 'NONE', #9102, #13572, #6324 ) ;
#9389=LINE ( 'NONE', #12080, #14947 ) ;
#9390=EDGE_CURVE ( 'NONE', #17860, #16352, #15944, .T. ) ;
#9415=DIRECTION ( 'NONE',  ( 1.224646799147350002E-16, -1.000000000000000000, -6.123233995736769734E-17 ) ) ;
#9424=VECTOR ( 'NONE', #9642, 1000.000000000000000 ) ;
#9489=EDGE_CURVE ( 'NONE', #8884, #9633, #7820, .T. ) ;
#9527=EDGE_LOOP ( 'NONE', ( #4645, #18217, #7285, #17020 ) ) ;
#9536=ADVANCED_FACE ( 'NONE', ( #14958 ), #6420, .T. ) ;
#9537=DIRECTION ( 'NONE',  ( -0.7071067811865480168, -1.847167598451501182E-16, 0.7071067811865470176 ) ) ;
#9632=ORIENTED_EDGE ( 'NONE', *, *, #15381, .T. ) ;
#9633=VERTEX_POINT ( 'NONE', #14348 ) ;
#9642=DIRECTION ( 'NONE',  ( 1.224510688924809779E-16, -1.000000000000000000, -1.306144734853129823E-16 ) ) ;
#9668=CARTESIAN_POINT ( 'NONE',  ( -0.5500000000000000444, 6.450000000000000178, 3.200000000000000178 ) ) ;
#9680=CARTESIAN_POINT ( 'NONE',  ( 0.2335786437626899970, 6.450000000000000178, 1.958578643762689753 ) ) ;
#9689=CARTESIAN_POINT ( 'NONE',  ( -0.3750000000000000000, 3.050000000000000266, 2.100000000000000089 ) ) ;
#9695=CARTESIAN_POINT ( 'NONE',  ( -0.3042893218813459977, 6.450000000000000178, 2.029289321881350361 ) ) ;
#9715=EDGE_CURVE ( 'NONE', #9633, #3220, #8706, .T. ) ;
#9733=ORIENTED_EDGE ( 'NONE', *, *, #1598, .T. ) ;
#9745=ADVANCED_FACE ( 'NONE', ( #6100 ), #11763, .F. ) ;
#9765=VECTOR ( 'NONE', #100, 1000.000000000000000 ) ;
#9778=VECTOR ( 'NONE', #10232, 1000.000000000000000 ) ;
#9789=CARTESIAN_POINT ( 'NONE',  ( 0.5500000000000000444, 6.450000000000000178, 2.699264068711930253 ) ) ;
#9803=ORIENTED_EDGE ( 'NONE', *, *, #1896, .F. ) ;
#9829=DIRECTION ( 'NONE',  ( 1.306144734853129823E-16, -1.000000000000000000, 0.000000000000000000 ) ) ;
#9844=CARTESIAN_POINT ( 'NONE',  ( 0.5500000000000000444, 3.050000000000000266, 3.399999999999999911 ) ) ;
#9850=EDGE_CURVE ( 'NONE', #9328, #8832, #2942, .T. ) ;
#9872=ORIENTED_EDGE ( 'NONE', *, *, #9390, .T. ) ;
#9873=EDGE_CURVE ( 'NONE', #7939, #11433, #10919, .T. ) ;
#9896=ORIENTED_EDGE ( 'NONE', *, *, #13790, .F. ) ;
#9944=ORIENTED_EDGE ( 'NONE', *, *, #6476, .F. ) ;
#9945=ADVANCED_FACE ( 'NONE', ( #6808 ), #14019, .T. ) ;
#9957=CIRCLE ( 'NONE', #4325, 0.1999999999999999833 ) ;
#10007=AXIS2_PLACEMENT_3D ( 'NONE', #2772, #166, #4323 ) ;
#10011=ORIENTED_EDGE ( 'NONE', *, *, #4924, .T. ) ;
#10028=DIRECTION ( 'NONE',  ( -1.000000000000000000, 0.000000000000000000, 0.000000000000000000 ) ) ;
#10032=ORIENTED_EDGE ( 'NONE', *, *, #8470, .T. ) ;
#10045=CARTESIAN_POINT ( 'NONE',  ( -0.5500000000000000444, 3.050000000000000266, 3.299999999999999822 ) ) ;
#10049=ORIENTED_EDGE ( 'NONE', *, *, #5746, .T. ) ;
#10052=ORIENTED_EDGE ( 'NONE', *, *, #15933, .F. ) ;
#10062=CARTESIAN_POINT ( 'NONE',  ( 0.7500000000000000000, 3.050000000000000266, 2.699264068711930253 ) ) ;
#10082=CARTESIAN_POINT ( 'NONE',  ( -0.6914213562373099364, 6.450000000000000178, 2.557842712474620139 ) ) ;
#10085=AXIS2_PLACEMENT_3D ( 'NONE', #9680, #1174, #4213 ) ;
#10088=LINE ( 'NONE', #7400, #7606 ) ;
#10115=EDGE_LOOP ( 'NONE', ( #10730, #16198, #18122, #3421, #17010, #2964, #15461, #3781, #6396, #72, #7091, #3702, #9083, #7717, #18061, #12478, #9944, #2239, #8998, #17076, #3907, #17618, #7614, #5096, #8668, #1387, #1248, #10201 ) ) ;
#10124=ORIENTED_EDGE ( 'NONE', *, *, #10322, .T. ) ;
#10138=VERTEX_POINT ( 'NONE', #12613 ) ;
#10141=DIRECTION ( 'NONE',  ( -0.7071067811865480168, 0.000000000000000000, 0.7071067811865470176 ) ) ;
#10155=ORIENTED_EDGE ( 'NONE', *, *, #4749, .T. ) ;
#10159=ORIENTED_EDGE ( 'NONE', *, *, #17493, .F. ) ;
#10181=CARTESIAN_POINT ( 'NONE',  ( 0.3042893218813439438, 6.450000000000000178, 2.170710678118660031 ) ) ;
#10185=EDGE_CURVE ( 'NONE', #12466, #14118, #18236, .T. ) ;
#10201=ORIENTED_EDGE ( 'NONE', *, *, #12205, .F. ) ;
#10224=VECTOR ( 'NONE', #11, 1000.000000000000000 ) ;
#10232=DIRECTION ( 'NONE',  ( 0.7071067811865470176, 0.000000000000000000, -0.7071067811865480168 ) ) ;
#10265=VECTOR ( 'NONE', #206, 1000.000000000000000 ) ;
#10272=AXIS2_PLACEMENT_3D ( 'NONE', #3735, #17707, #886 ) ;
#10306=VECTOR ( 'NONE', #7806, 1000.000000000000114 ) ;
#10322=EDGE_CURVE ( 'NONE', #12793, #17050, #4897, .T. ) ;
#10326=LINE ( 'NONE', #13185, #771 ) ;
#10329=CARTESIAN_POINT ( 'NONE',  ( -0.3042893218813459977, 3.050000000000000266, 2.029289321881350361 ) ) ;
#10340=DIRECTION ( 'NONE',  ( 1.632680918566409751E-16, -1.000000000000000000, 0.000000000000000000 ) ) ;
#10358=DIRECTION ( 'NONE',  ( 1.306144734853129823E-16, -1.000000000000000000, 0.000000000000000000 ) ) ;
#10359=AXIS2_PLACEMENT_3D ( 'NONE', #12676, #18106, #16835 ) ;
#10366=VECTOR ( 'NONE', #16678, 1000.000000000000000 ) ;
#10398=CARTESIAN_POINT ( 'NONE',  ( 0.5921572875253799939, 3.050000000000000266, 1.600000000000000089 ) ) ;
#10405=CARTESIAN_POINT ( 'NONE',  ( -0.6500000000000000222, 6.450000000000000178, 2.699264068711930253 ) ) ;
#10423=DIRECTION ( 'NONE',  ( 0.7071067811865489050, 0.000000000000000000, 0.7071067811865460184 ) ) ;
#10434=AXIS2_PLACEMENT_3D ( 'NONE', #6270, #13407, #13502 ) ;
#10440=VECTOR ( 'NONE', #18140, 1000.000000000000000 ) ;
#10445=EDGE_LOOP ( 'NONE', ( #2941, #1147, #10159, #8077 ) ) ;
#10469=ORIENTED_EDGE ( 'NONE', *, *, #1258, .T. ) ;
#10503=CARTESIAN_POINT ( 'NONE',  ( -0.6628679656440369383, 6.450000000000000178, 1.670710678118660031 ) ) ;
#10506=ORIENTED_EDGE ( 'NONE', *, *, #17058, .T. ) ;
#10516=AXIS2_PLACEMENT_3D ( 'NONE', #8975, #1676, #382 ) ;
#10524=CARTESIAN_POINT ( 'NONE',  ( 0.6628679656440349399, 3.050000000000000266, 1.670710678118660031 ) ) ;
#10526=CLOSED_SHELL ( 'NONE', ( #9745, #11186, #12492, #7686, #1213, #4360, #12535, #14753, #3386, #16575, #2512, #10883, #9945, #3984, #11730, #15817, #7953, #561, #11947, #15146, #16516, #9536, #16848, #13331, #6523, #3153, #3262, #3459, #11920, #472 ) ) ;
#10559=CIRCLE ( 'NONE', #3186, 0.2000000000000000389 ) ;
#10573=EDGE_LOOP ( 'NONE', ( #9169, #12078, #10776, #706 ) ) ;
#10604=FACE_OUTER_BOUND ( 'NONE', #164, .T. ) ;
#10605=LINE ( 'NONE', #11130, #10440 ) ;
#10613=EDGE_CURVE ( 'NONE', #2304, #5170, #16855, .T. ) ;
#10647=VECTOR ( 'NONE', #9142, 1000.000000000000000 ) ;
#10670=PRODUCT_DEFINITION_SHAPE ( 'NONE', 'NONE',  #15932 ) ;
#10677=ORIENTED_EDGE ( 'NONE', *, *, #9002, .T. ) ;
#10706=VERTEX_POINT ( 'NONE', #10524 ) ;
#10713=DIRECTION ( 'NONE',  ( 1.000000000000000000, 0.000000000000000000, 0.000000000000000000 ) ) ;
#10730=ORIENTED_EDGE ( 'NONE', *, *, #9489, .F. ) ;
#10773=DIRECTION ( 'NONE',  ( 4.898042755699219270E-17, -1.000000000000000000, 0.000000000000000000 ) ) ;
#10776=ORIENTED_EDGE ( 'NONE', *, *, #16148, .F. ) ;
#10784=DIRECTION ( 'NONE',  ( -1.224646799147351975E-16, 1.000000000000000000, 6.123233995736759873E-17 ) ) ;
#10796=ORIENTED_EDGE ( 'NONE', *, *, #12779, .T. ) ;
#10798=CARTESIAN_POINT ( 'NONE',  ( 0.6914213562373080491, 6.450000000000000178, 2.557842712474620139 ) ) ;
#10836=VECTOR ( 'NONE', #17229, 1000.000000000000114 ) ;
#10846=EDGE_CURVE ( 'NONE', #14829, #12759, #17382, .T. ) ;
#10875=ORIENTED_EDGE ( 'NONE', *, *, #12357, .T. ) ;
#10881=CYLINDRICAL_SURFACE ( 'NONE', #10272, 0.1000000000000000472 ) ;
#10883=ADVANCED_FACE ( 'NONE', ( #16567 ), #10922, .F. ) ;
#10894=DIRECTION ( 'NONE',  ( -1.000000000000000000, 0.000000000000000000, 0.000000000000000000 ) ) ;
#10919=CIRCLE ( 'NONE', #13270, 0.1000000000000000472 ) ;
#10922=CYLINDRICAL_SURFACE ( 'NONE', #8579, 0.1000000000000001443 ) ;
#10979=DIRECTION ( 'NONE',  ( 1.306144734853129823E-16, -1.000000000000000000, 0.000000000000000000 ) ) ;
#10992=ORIENTED_EDGE ( 'NONE', *, *, #5746, .F. ) ;
#10999=EDGE_CURVE ( 'NONE', #8884, #16183, #16654, .T. ) ;
#11019=FACE_OUTER_BOUND ( 'NONE', #16304, .T. ) ;
#11024=VECTOR ( 'NONE', #9196, 1000.000000000000000 ) ;
#11030=LINE ( 'NONE', #8166, #12755 ) ;
#11057=CIRCLE ( 'NONE', #14312, 0.2000000000000000389 ) ;
#11075=VERTEX_POINT ( 'NONE', #13505 ) ;
#11092=ORIENTED_EDGE ( 'NONE', *, *, #2728, .F. ) ;
#11093=DIRECTION ( 'NONE',  ( -0.7071067811865475727, -2.050767998142408981E-32, -0.7071067811865475727 ) ) ;
#11094=FACE_OUTER_BOUND ( 'NONE', #13173, .T. ) ;
#11101=FACE_OUTER_BOUND ( 'NONE', #13161, .T. ) ;
#11103=CARTESIAN_POINT ( 'NONE',  ( -0.3750000000000000000, 6.450000000000000178, 2.100000000000000089 ) ) ;
#11124=CARTESIAN_POINT ( 'NONE',  ( 0.5500000000000000444, 6.450000000000000178, 3.299999999999999822 ) ) ;
#11130=CARTESIAN_POINT ( 'NONE',  ( 0.3042893218813439438, 6.450000000000000178, 2.029289321881350361 ) ) ;
#11151=DIRECTION ( 'NONE',  ( -0.7071067811865470176, -9.235837992257497283E-17, 0.7071067811865480168 ) ) ;
#11163=FACE_OUTER_BOUND ( 'NONE', #3673, .T. ) ;
#11186=ADVANCED_FACE ( 'NONE', ( #4141 ), #15459, .T. ) ;
#11191=CARTESIAN_POINT ( 'NONE',  ( 0.000000000000000000, 0.000000000000000000, 0.000000000000000000 ) ) ;
#11249=DIRECTION ( 'NONE',  ( 1.224646799147350002E-16, -1.000000000000000000, -6.123233995736769734E-17 ) ) ;
#11267=CARTESIAN_POINT ( 'NONE',  ( 0.7500000000000000000, 6.450000000000000178, 2.699264068711930253 ) ) ;
#11292=CARTESIAN_POINT ( 'NONE',  ( -0.5500000000000000444, 3.050000000000000266, 2.699264068711930253 ) ) ;
#11295=DIRECTION ( 'NONE',  ( -0.7071067811865480168, 0.000000000000000000, -0.7071067811865470176 ) ) ;
#11329=ORIENTED_EDGE ( 'NONE', *, *, #15495, .T. ) ;
#11332=EDGE_CURVE ( 'NONE', #6891, #12909, #4720, .T. ) ;
#11340=LINE ( 'NONE', #5959, #10836 ) ;
#11361=DIRECTION ( 'NONE',  ( 1.224646799147350002E-16, -1.000000000000000000, -6.123233995736779594E-17 ) ) ;
#11379=DIRECTION ( 'NONE',  ( -1.000000000000000000, 0.000000000000000000, 0.000000000000000000 ) ) ;
#11382=LINE ( 'NONE', #1378, #11729 ) ;
#11410=EDGE_CURVE ( 'NONE', #16183, #3220, #4683, .T. ) ;
#11413=EDGE_CURVE ( 'NONE', #9351, #11433, #7649, .T. ) ;
#11433=VERTEX_POINT ( 'NONE', #433 ) ;
#11456=DIRECTION ( 'NONE',  ( 0.000000000000000000, 6.123233995736769734E-17, -1.000000000000000000 ) ) ;
#11461=PLANE ( 'NONE',  #6528 ) ;
#11507=EDGE_LOOP ( 'NONE', ( #15187, #7989, #10506, #12941, #8729, #14812, #7620, #16498, #353, #11617, #10155, #18109, #9872, #18040, #10011, #6289, #18272, #15134, #7991, #6739, #9733, #258, #15393, #5102, #13637, #1892, #18141, #17093 ) ) ;
#11508=VECTOR ( 'NONE', #554, 1000.000000000000000 ) ;
#11520=VECTOR ( 'NONE', #4721, 1000.000000000000000 ) ;
#11523=LINE ( 'NONE', #17151, #11905 ) ;
#11534=EDGE_CURVE ( 'NONE', #6673, #12793, #17900, .T. ) ;
#11562=CARTESIAN_POINT ( 'NONE',  ( -0.5500000000000000444, 6.450000000000000178, 3.399999999999999911 ) ) ;
#11569=EDGE_CURVE ( 'NONE', #5150, #6699, #4953, .T. ) ;
#11582=CARTESIAN_POINT ( 'NONE',  ( -0.7500000000000000000, 6.450000000000000178, 2.699264068711930253 ) ) ;
#11608=EDGE_LOOP ( 'NONE', ( #9632, #15524, #6123, #14530 ) ) ;
#11617=ORIENTED_EDGE ( 'NONE', *, *, #16963, .T. ) ;
#11622=DIRECTION ( 'NONE',  ( 0.7071067811865594521, 0.000000000000000000, 0.7071067811865355823 ) ) ;
#11725=CARTESIAN_POINT ( 'NONE',  ( -0.5921572875253819923, 6.450000000000000178, 1.600000000000000089 ) ) ;
#11726=SHAPE_REPRESENTATION_RELATIONSHIP ( 'NONE' , 'NONE' ,  #4614, #686 ) ;
#11729=VECTOR ( 'NONE', #11295, 1000.000000000000000 ) ;
#11730=ADVANCED_FACE ( 'NONE', ( #7532 ), #15709, .T. ) ;
#11739=CIRCLE ( 'NONE', #8777, 0.09999999999999982514 ) ;
#11758=CARTESIAN_POINT ( 'NONE',  ( -0.6914213562373099364, 3.050000000000000266, 2.557842712474620139 ) ) ;
#11760=CIRCLE ( 'NONE', #1984, 0.2000000000000000944 ) ;
#11762=EDGE_CURVE ( 'NONE', #2304, #16266, #17156, .T. ) ;
#11763=PLANE ( 'NONE',  #7960 ) ;
#11766=FILL_AREA_STYLE_COLOUR ( '', #5835 ) ;
#11783=EDGE_LOOP ( 'NONE', ( #2384, #7443, #2432, #19 ) ) ;
#11818=ORIENTED_EDGE ( 'NONE', *, *, #340, .F. ) ;
#11834=CARTESIAN_POINT ( 'NONE',  ( -4.163799117100999573E-16, 6.450000000000000178, 3.949485927250209908E-16 ) ) ;
#11840=CARTESIAN_POINT ( 'NONE',  ( -0.3042893218813459977, 3.050000000000000266, 2.029289321881350361 ) ) ;
#11850=AXIS2_PLACEMENT_3D ( 'NONE', #1996, #9415, #5244 ) ;
#11875=EDGE_LOOP ( 'NONE', ( #314, #8484, #1283, #8981 ) ) ;
#11898=DIRECTION ( 'NONE',  ( -1.000000000000000000, 0.000000000000000000, 0.000000000000000000 ) ) ;
#11905=VECTOR ( 'NONE', #5786, 1000.000000000000000 ) ;
#11920=ADVANCED_FACE ( 'NONE', ( #16738 ), #17095, .T. ) ;
#11947=ADVANCED_FACE ( 'NONE', ( #12769 ), #11461, .T. ) ;
#11955=ORIENTED_EDGE ( 'NONE', *, *, #12876, .F. ) ;
#11956=CARTESIAN_POINT ( 'NONE',  ( 0.3750000000000000000, 6.450000000000000178, 2.100000000000000089 ) ) ;
#11985=LINE ( 'NONE', #4939, #2154 ) ;
#11989=DIRECTION ( 'NONE',  ( 1.224646799147350002E-16, -1.000000000000000000, -6.123233995736769734E-17 ) ) ;
#12031=EDGE_LOOP ( 'NONE', ( #3559, #16193, #12704, #1324 ) ) ;
#12039=VECTOR ( 'NONE', #5933, 1000.000000000000000 ) ;
#12051=ORIENTED_EDGE ( 'NONE', *, *, #11410, .F. ) ;
#12078=ORIENTED_EDGE ( 'NONE', *, *, #12220, .T. ) ;
#12080=CARTESIAN_POINT ( 'NONE',  ( 0.6207106781186549904, 3.050000000000000266, 2.628553390593269423 ) ) ;
#12107=AXIS2_PLACEMENT_3D ( 'NONE', #7749, #16449, #8046 ) ;
#12109=EDGE_CURVE ( 'NONE', #6911, #9328, #6255, .T. ) ;
#12115=LINE ( 'NONE', #2005, #5276 ) ;
#12176=FACE_OUTER_BOUND ( 'NONE', #11875, .T. ) ;
#12193=ORIENTED_EDGE ( 'NONE', *, *, #16713, .F. ) ;
#12205=EDGE_CURVE ( 'NONE', #9633, #14829, #269, .T. ) ;
#12210=DIRECTION ( 'NONE',  ( 0.000000000000000000, 0.000000000000000000, -1.000000000000000000 ) ) ;
#12217=ORIENTED_EDGE ( 'NONE', *, *, #6476, .T. ) ;
#12220=EDGE_CURVE ( 'NONE', #12458, #14546, #4687, .T. ) ;
#12241=CARTESIAN_POINT ( 'NONE',  ( 0.3042893218813439438, 6.450000000000000178, 2.029289321881350361 ) ) ;
#12249=EDGE_CURVE ( 'NONE', #3809, #16824, #606, .T. ) ;
#12265=LINE ( 'NONE', #10405, #3147 ) ;
#12269=PLANE ( 'NONE',  #9374 ) ;
#12273=CARTESIAN_POINT ( 'NONE',  ( -0.7500000000000000000, 3.050000000000000266, 2.699264068711930253 ) ) ;
#12278=FACE_OUTER_BOUND ( 'NONE', #2558, .T. ) ;
#12283=DIRECTION ( 'NONE',  ( 0.000000000000000000, 0.000000000000000000, -1.000000000000000000 ) ) ;
#12307=DIRECTION ( 'NONE',  ( 0.7071067811865489050, 0.000000000000000000, -0.7071067811865461294 ) ) ;
#12357=EDGE_CURVE ( 'NONE', #10138, #9165, #1079, .T. ) ;
#12367=CARTESIAN_POINT ( 'NONE',  ( 0.5500000000000000444, 6.450000000000000178, 3.399999999999999911 ) ) ;
#12444=LINE ( 'NONE', #16787, #5870 ) ;
#12458=VERTEX_POINT ( 'NONE', #10798 ) ;
#12466=VERTEX_POINT ( 'NONE', #4125 ) ;
#12478=ORIENTED_EDGE ( 'NONE', *, *, #4216, .F. ) ;
#12492=ADVANCED_FACE ( 'NONE', ( #63 ), #12748, .T. ) ;
#12501=CARTESIAN_POINT ( 'NONE',  ( 0.5921572875253799939, 6.450000000000000178, 1.600000000000000089 ) ) ;
#12535=ADVANCED_FACE ( 'NONE', ( #11163 ), #2656, .T. ) ;
#12549=PLANE ( 'NONE',  #968 ) ;
#12589=ORIENTED_EDGE ( 'NONE', *, *, #12760, .F. ) ;
#12602=CYLINDRICAL_SURFACE ( 'NONE', #1982, 0.2000000000000000389 ) ;
#12613=CARTESIAN_POINT ( 'NONE',  ( 0.6500000000000000222, 6.450000000000000178, 3.200000000000000178 ) ) ;
#12660=DIRECTION ( 'NONE',  ( 0.000000000000000000, 0.000000000000000000, 1.000000000000000000 ) ) ;
#12671=CARTESIAN_POINT ( 'NONE',  ( 0.000000000000000000, 3.050000000000000266, 1.867586368699710122E-16 ) ) ;
#12674=EDGE_CURVE ( 'NONE', #6214, #9105, #3541, .T. ) ;
#12676=CARTESIAN_POINT ( 'NONE',  ( 0.6628679656440349399, 6.450000000000000178, 1.670710678118660031 ) ) ;
#12704=ORIENTED_EDGE ( 'NONE', *, *, #15794, .F. ) ;
#12705=AXIS2_PLACEMENT_3D ( 'NONE', #13745, #1251, #15338 ) ;
#12748=PLANE ( 'NONE',  #10085 ) ;
#12754=FACE_OUTER_BOUND ( 'NONE', #12031, .T. ) ;
#12755=VECTOR ( 'NONE', #9829, 1000.000000000000000 ) ;
#12759=VERTEX_POINT ( 'NONE', #12241 ) ;
#12760=EDGE_CURVE ( 'NONE', #14294, #12466, #7718, .T. ) ;
#12761=CYLINDRICAL_SURFACE ( 'NONE', #16803, 0.1999999999999999833 ) ;
#12769=FACE_OUTER_BOUND ( 'NONE', #8287, .T. ) ;
#12771=ORIENTED_EDGE ( 'NONE', *, *, #9715, .F. ) ;
#12779=EDGE_CURVE ( 'NONE', #16312, #5150, #7701, .T. ) ;
#12788=CARTESIAN_POINT ( 'NONE',  ( -0.5500000000000000444, 6.450000000000000178, 3.299999999999999822 ) ) ;
#12793=VERTEX_POINT ( 'NONE', #14833 ) ;
#12797=CARTESIAN_POINT ( 'NONE',  ( -0.3750000000000000000, 6.450000000000000178, 2.100000000000000089 ) ) ;
#12813=EDGE_CURVE ( 'NONE', #14829, #10706, #7792, .T. ) ;
#12874=EDGE_CURVE ( 'NONE', #5170, #4541, #6951, .T. ) ;
#12876=EDGE_CURVE ( 'NONE', #6139, #14118, #11030, .T. ) ;
#12889=LINE ( 'NONE', #3154, #10265 ) ;
#12909=VERTEX_POINT ( 'NONE', #2438 ) ;
#12915=DIRECTION ( 'NONE',  ( 0.7071067811865480168, 9.235837992257497283E-17, -0.7071067811865470176 ) ) ;
#12939=VECTOR ( 'NONE', #10979, 1000.000000000000000 ) ;
#12941=ORIENTED_EDGE ( 'NONE', *, *, #16148, .T. ) ;
#12944=ORIENTED_EDGE ( 'NONE', *, *, #4865, .F. ) ;
#12990=ORIENTED_EDGE ( 'NONE', *, *, #1598, .F. ) ;
#13060=SURFACE_STYLE_USAGE ( .BOTH. , #8887 ) ;
#13106=ORIENTED_EDGE ( 'NONE', *, *, #9489, .T. ) ;
#13115=CIRCLE ( 'NONE', #6903, 0.1000000000000000472 ) ;
#13149=CARTESIAN_POINT ( 'NONE',  ( -0.5500000000000000444, 3.050000000000000266, 3.399999999999999911 ) ) ;
#13161=EDGE_LOOP ( 'NONE', ( #8211, #7674, #14382, #16793 ) ) ;
#13168=EDGE_CURVE ( 'NONE', #13931, #7939, #5072, .T. ) ;
#13173=EDGE_LOOP ( 'NONE', ( #16698, #1199, #16628, #10992 ) ) ;
#13185=CARTESIAN_POINT ( 'NONE',  ( -0.2335786437626909962, 6.450000000000000178, 2.241421356237310203 ) ) ;
#13194=CARTESIAN_POINT ( 'NONE',  ( -0.2335786437626909962, 3.050000000000000266, 2.241421356237310203 ) ) ;
#13200=DIRECTION ( 'NONE',  ( -0.7071067811865502373, 0.000000000000000000, -0.7071067811865447972 ) ) ;
#13230=VECTOR ( 'NONE', #7071, 1000.000000000000000 ) ;
#13247=AXIS2_PLACEMENT_3D ( 'NONE', #12797, #1596, #7240 ) ;
#13257=VECTOR ( 'NONE', #7469, 1000.000000000000000 ) ;
#13270=AXIS2_PLACEMENT_3D ( 'NONE', #2397, #13302, #10713 ) ;
#13285=DIRECTION ( 'NONE',  ( -0.7071067811865502373, 0.000000000000000000, -0.7071067811865447972 ) ) ;
#13302=DIRECTION ( 'NONE',  ( -1.224646799147350002E-16, 1.000000000000000000, 6.123233995736759873E-17 ) ) ;
#13306=CARTESIAN_POINT ( 'NONE',  ( 0.6914213562373089372, 3.050000000000000266, 2.557842712474620139 ) ) ;
#13308=AXIS2_PLACEMENT_3D ( 'NONE', #1814, #12915, #143 ) ;
#13331=ADVANCED_FACE ( 'NONE', ( #1465 ), #12761, .T. ) ;
#13384=DIRECTION ( 'NONE',  ( 0.000000000000000000, 0.000000000000000000, -1.000000000000000000 ) ) ;
#13407=DIRECTION ( 'NONE',  ( 1.000000000000000000, 1.306144734853129823E-16, 0.000000000000000000 ) ) ;
#13442=PRODUCT_CONTEXT ( 'NONE', #14650, 'mechanical' ) ;
#13475=DIRECTION ( 'NONE',  ( -0.7071067811865500152, 0.000000000000000000, -0.7071067811865451302 ) ) ;
#13483=DIRECTION ( 'NONE',  ( 0.000000000000000000, 0.000000000000000000, 1.000000000000000000 ) ) ;
#13502=DIRECTION ( 'NONE',  ( -1.306144734853129823E-16, 1.000000000000000000, 0.000000000000000000 ) ) ;
#13505=CARTESIAN_POINT ( 'NONE',  ( -0.3042893218813459977, 6.450000000000000178, 2.170710678118660031 ) ) ;
#13522=DIRECTION ( 'NONE',  ( 0.000000000000000000, -1.000000000000000000, -1.959217102279674889E-16 ) ) ;
#13523=AXIS2_PLACEMENT_3D ( 'NONE', #2386, #2469, #13475 ) ;
#13532=ORIENTED_EDGE ( 'NONE', *, *, #322, .F. ) ;
#13537=DIRECTION ( 'NONE',  ( 1.000000000000000000, 0.000000000000000000, 0.000000000000000000 ) ) ;
#13566=EDGE_CURVE ( 'NONE', #8965, #6891, #16075, .T. ) ;
#13572=DIRECTION ( 'NONE',  ( -1.000000000000000000, -1.306144734853129823E-16, 0.000000000000000000 ) ) ;
#13618=AXIS2_PLACEMENT_3D ( 'NONE', #7390, #7473, #13200 ) ;
#13637=ORIENTED_EDGE ( 'NONE', *, *, #9873, .T. ) ;
#13657=DIRECTION ( 'NONE',  ( 9.796085511398438540E-17, -1.000000000000000000, -6.530723674265629391E-17 ) ) ;
#13673=CARTESIAN_POINT ( 'NONE',  ( -0.7500000000000000000, 6.450000000000000178, 3.200000000000000178 ) ) ;
#13713=DIRECTION ( 'NONE',  ( 0.7071067811865461294, 1.385375698838618738E-16, -0.7071067811865490160 ) ) ;
#13745=CARTESIAN_POINT ( 'NONE',  ( -0.2335786437626909962, 6.450000000000000178, 2.241421356237310203 ) ) ;
#13748=EDGE_LOOP ( 'NONE', ( #9372, #10032, #12589, #7099 ) ) ;
#13790=EDGE_CURVE ( 'NONE', #11075, #17860, #6140, .T. ) ;
#13865=DIRECTION ( 'NONE',  ( -1.224646799147350002E-16, 1.000000000000000000, 6.123233995736759873E-17 ) ) ;
#13868=CARTESIAN_POINT ( 'NONE',  ( -0.6500000000000000222, 6.450000000000000178, 3.200000000000000178 ) ) ;
#13876=DIRECTION ( 'NONE',  ( 1.224646799147350002E-16, -1.000000000000000000, -6.123233995736769734E-17 ) ) ;
#13931=VERTEX_POINT ( 'NONE', #13990 ) ;
#13936=DIRECTION ( 'NONE',  ( 1.000000000000000000, 0.000000000000000000, 0.000000000000000000 ) ) ;
#13945=EDGE_LOOP ( 'NONE', ( #13106, #14049, #12051, #3414 ) ) ;
#13955=DIRECTION ( 'NONE',  ( 0.7071067811865480168, 0.000000000000000000, 0.7071067811865470176 ) ) ;
#13967=EDGE_CURVE ( 'NONE', #6214, #8884, #1402, .T. ) ;
#13989=FACE_OUTER_BOUND ( 'NONE', #10445, .T. ) ;
#13990=CARTESIAN_POINT ( 'NONE',  ( 0.6500000000000000222, 3.050000000000000266, 3.200000000000000178 ) ) ;
#13993=CARTESIAN_POINT ( 'NONE',  ( 0.5921572875253799939, 3.050000000000000266, 1.600000000000000089 ) ) ;
#14019=PLANE ( 'NONE',  #12705 ) ;
#14021=PLANE ( 'NONE',  #7027 ) ;
#14028=ORIENTED_EDGE ( 'NONE', *, *, #3238, .T. ) ;
#14049=ORIENTED_EDGE ( 'NONE', *, *, #9715, .T. ) ;
#14064=CARTESIAN_POINT ( 'NONE',  ( 0.2335786437626899970, 6.450000000000000178, 2.241421356237310203 ) ) ;
#14101=EDGE_CURVE ( 'NONE', #9239, #6891, #14452, .T. ) ;
#14118=VERTEX_POINT ( 'NONE', #13149 ) ;
#14177=VERTEX_POINT ( 'NONE', #4153 ) ;
#14191=LINE ( 'NONE', #11124, #13230 ) ;
#14294=VERTEX_POINT ( 'NONE', #8775 ) ;
#14296=ORIENTED_EDGE ( 'NONE', *, *, #4216, .T. ) ;
#14312=AXIS2_PLACEMENT_3D ( 'NONE', #1587, #5831, #14342 ) ;
#14331=EDGE_CURVE ( 'NONE', #16312, #16352, #10088, .T. ) ;
#14338=CARTESIAN_POINT ( 'NONE',  ( -0.6500000000000000222, 6.450000000000000178, 3.200000000000000178 ) ) ;
#14342=DIRECTION ( 'NONE',  ( 0.7071067811865466846, 0.000000000000000000, -0.7071067811865483499 ) ) ;
#14348=CARTESIAN_POINT ( 'NONE',  ( 0.5921572875253799939, 6.450000000000000178, 1.600000000000000089 ) ) ;
#14354=CYLINDRICAL_SURFACE ( 'NONE', #10516, 0.1000000000000000472 ) ;
#14356=CYLINDRICAL_SURFACE ( 'NONE', #14408, 0.2000000000000000389 ) ;
#14357=CARTESIAN_POINT ( 'NONE',  ( 0.6500000000000000222, 6.450000000000000178, 2.699264068711930253 ) ) ;
#14382=ORIENTED_EDGE ( 'NONE', *, *, #4924, .F. ) ;
#14408=AXIS2_PLACEMENT_3D ( 'NONE', #2895, #5675, #5760 ) ;
#14452=LINE ( 'NONE', #3406, #12039 ) ;
#14457=CARTESIAN_POINT ( 'NONE',  ( -0.6914213562373099364, 6.450000000000000178, 2.557842712474620139 ) ) ;
#14483=VECTOR ( 'NONE', #10028, 1000.000000000000000 ) ;
#14511=EDGE_LOOP ( 'NONE', ( #14811, #16983, #16026, #15877 ) ) ;
#14530=ORIENTED_EDGE ( 'NONE', *, *, #15192, .F. ) ;
#14546=VERTEX_POINT ( 'NONE', #13306 ) ;
#14552=DIRECTION ( 'NONE',  ( -1.224646799147351975E-16, 1.000000000000000000, 6.123233995736759873E-17 ) ) ;
#14600=EDGE_CURVE ( 'NONE', #14177, #8965, #10559, .T. ) ;
#14633=DIRECTION ( 'NONE',  ( -0.7071067811865500152, 0.000000000000000000, -0.7071067811865451302 ) ) ;
#14650=APPLICATION_CONTEXT ( 'automotive_design' ) ;
#14653=EDGE_CURVE ( 'NONE', #7292, #268, #8129, .T. ) ;
#14682=CIRCLE ( 'NONE', #218, 0.09999999999999982514 ) ;
#14702=ORIENTED_EDGE ( 'NONE', *, *, #15495, .F. ) ;
#14712=EDGE_CURVE ( 'NONE', #9165, #9351, #1118, .T. ) ;
#14731=DIRECTION ( 'NONE',  ( 1.306144734853129823E-16, -1.000000000000000000, -6.530723674265629391E-17 ) ) ;
#14741=CARTESIAN_POINT ( 'NONE',  ( 0.5500000000000000444, 6.450000000000000178, 2.699264068711930253 ) ) ;
#14753=ADVANCED_FACE ( 'NONE', ( #12754 ), #4220, .F. ) ;
#14762=CARTESIAN_POINT ( 'NONE',  ( -0.5500000000000000444, 6.450000000000000178, 2.699264068711930253 ) ) ;
#14811=ORIENTED_EDGE ( 'NONE', *, *, #16562, .T. ) ;
#14812=ORIENTED_EDGE ( 'NONE', *, *, #7123, .T. ) ;
#14829=VERTEX_POINT ( 'NONE', #4487 ) ;
#14833=CARTESIAN_POINT ( 'NONE',  ( -0.7500000000000000000, 6.450000000000000178, 2.699264068711930253 ) ) ;
#14840=EDGE_CURVE ( 'NONE', #8832, #9239, #10326, .T. ) ;
#14852=CARTESIAN_POINT ( 'NONE',  ( 0.2335786437626899970, 6.450000000000000178, 2.241421356237310203 ) ) ;
#14895=PLANE ( 'NONE',  #10434 ) ;
#14947=VECTOR ( 'NONE', #2364, 1000.000000000000000 ) ;
#14958=FACE_OUTER_BOUND ( 'NONE', #8599, .T. ) ;
#14963=CARTESIAN_POINT ( 'NONE',  ( 0.3750000000000000000, 3.050000000000000266, 2.100000000000000089 ) ) ;
#14992=CARTESIAN_POINT ( 'NONE',  ( 0.6500000000000000222, 3.050000000000000266, 3.200000000000000178 ) ) ;
#15134=ORIENTED_EDGE ( 'NONE', *, *, #13566, .T. ) ;
#15146=ADVANCED_FACE ( 'NONE', ( #12176 ), #2174, .T. ) ;
#15187=ORIENTED_EDGE ( 'NONE', *, *, #17726, .T. ) ;
#15192=EDGE_CURVE ( 'NONE', #2742, #12909, #12265, .T. ) ;
#15240=AXIS2_PLACEMENT_3D ( 'NONE', #11292, #16929, #11379 ) ;
#15315=( GEOMETRIC_REPRESENTATION_CONTEXT ( 3 ) GLOBAL_UNCERTAINTY_ASSIGNED_CONTEXT ( ( #1038 ) ) GLOBAL_UNIT_ASSIGNED_CONTEXT ( ( #15942, #16028, #4446 ) ) REPRESENTATION_CONTEXT ( 'NONE', 'WORKASPACE' ) );
#15325=CARTESIAN_POINT ( 'NONE',  ( -0.3042893218813459977, 3.050000000000000266, 2.170710678118660031 ) ) ;
#15338=DIRECTION ( 'NONE',  ( -8.163404592832159998E-18, -1.000000000000000000, 0.000000000000000000 ) ) ;
#15340=LINE ( 'NONE', #2647, #12939 ) ;
#15381=EDGE_CURVE ( 'NONE', #2742, #9183, #15699, .T. ) ;
#15393=ORIENTED_EDGE ( 'NONE', *, *, #15794, .T. ) ;
#15410=FACE_OUTER_BOUND ( 'NONE', #9527, .T. ) ;
#15424=VECTOR ( 'NONE', #10423, 1000.000000000000114 ) ;
#15451=DIRECTION ( 'NONE',  ( 1.306144734853129823E-16, -1.000000000000000000, 0.000000000000000000 ) ) ;
#15459=PLANE ( 'NONE',  #6502 ) ;
#15461=ORIENTED_EDGE ( 'NONE', *, *, #11762, .F. ) ;
#15478=EDGE_CURVE ( 'NONE', #5150, #6911, #11340, .T. ) ;
#15495=EDGE_CURVE ( 'NONE', #9165, #7939, #17147, .T. ) ;
#15524=ORIENTED_EDGE ( 'NONE', *, *, #741, .T. ) ;
#15554=FACE_OUTER_BOUND ( 'NONE', #1881, .T. ) ;
#15602=EDGE_CURVE ( 'NONE', #12793, #8985, #9957, .T. ) ;
#15623=STYLED_ITEM ( 'NONE', ( #5839 ), #7724 ) ;
#15632=CIRCLE ( 'NONE', #5263, 0.09999999999999986677 ) ;
#15674=DIRECTION ( 'NONE',  ( 1.306144734853129823E-16, -1.000000000000000000, 0.000000000000000000 ) ) ;
#15688=ORIENTED_EDGE ( 'NONE', *, *, #13566, .F. ) ;
#15699=LINE ( 'NONE', #3180, #4034 ) ;
#15708=VECTOR ( 'NONE', #12283, 1000.000000000000000 ) ;
#15709=PLANE ( 'NONE',  #13308 ) ;
#15762=DIRECTION ( 'NONE',  ( -1.000000000000000000, 0.000000000000000000, 0.000000000000000000 ) ) ;
#15778=ORIENTED_EDGE ( 'NONE', *, *, #11534, .T. ) ;
#15794=EDGE_CURVE ( 'NONE', #4541, #13931, #14682, .T. ) ;
#15801=EDGE_CURVE ( 'NONE', #9351, #6214, #11382, .T. ) ;
#15817=ADVANCED_FACE ( 'NONE', ( #11101 ), #16846, .T. ) ;
#15826=DIRECTION ( 'NONE',  ( 0.7071067811865480168, 0.000000000000000000, 0.7071067811865470176 ) ) ;
#15847=CARTESIAN_POINT ( 'NONE',  ( -0.5500000000000000444, 6.450000000000000178, 3.200000000000000178 ) ) ;
#15877=ORIENTED_EDGE ( 'NONE', *, *, #14101, .F. ) ;
#15932=PRODUCT_DEFINITION ( 'UNKNOWN', '', #17414, #17859 ) ;
#15933=EDGE_CURVE ( 'NONE', #16352, #6699, #6184, .T. ) ;
#15942=( LENGTH_UNIT ( ) NAMED_UNIT ( * ) SI_UNIT ( .MILLI., .METRE. ) );
#15944=CIRCLE ( 'NONE', #4113, 0.09999999999999997780 ) ;
#15946=AXIS2_PLACEMENT_3D ( 'NONE', #15847, #15948, #15762 ) ;
#15948=DIRECTION ( 'NONE',  ( -1.224646799147350002E-16, 1.000000000000000000, 6.123233995736769734E-17 ) ) ;
#15993=VECTOR ( 'NONE', #7294, 1000.000000000000000 ) ;
#16000=CARTESIAN_POINT ( 'NONE',  ( 0.6207106781186539912, 6.450000000000000178, 2.628553390593269423 ) ) ;
#16026=ORIENTED_EDGE ( 'NONE', *, *, #11332, .F. ) ;
#16028=( NAMED_UNIT ( * ) PLANE_ANGLE_UNIT ( ) SI_UNIT ( $, .RADIAN. ) );
#16034=CARTESIAN_POINT ( 'NONE',  ( 0.3042893218813449985, 3.050000000000000266, 2.029289321881350361 ) ) ;
#16065=DIRECTION ( 'NONE',  ( 1.306144734853129823E-16, -1.000000000000000000, -1.306144734853129823E-16 ) ) ;
#16075=LINE ( 'NONE', #13194, #13257 ) ;
#16124=DIRECTION ( 'NONE',  ( -0.7071067811865470176, 0.000000000000000000, -0.7071067811865480168 ) ) ;
#16127=LINE ( 'NONE', #4909, #18231 ) ;
#16148=EDGE_CURVE ( 'NONE', #268, #14546, #8492, .T. ) ;
#16153=AXIS2_PLACEMENT_3D ( 'NONE', #6239, #683, #11898 ) ;
#16183=VERTEX_POINT ( 'NONE', #2664 ) ;
#16188=FACE_OUTER_BOUND ( 'NONE', #11608, .T. ) ;
#16193=ORIENTED_EDGE ( 'NONE', *, *, #16713, .T. ) ;
#16194=CARTESIAN_POINT ( 'NONE',  ( 0.7500000000000000000, 6.450000000000000178, 3.200000000000000178 ) ) ;
#16198=ORIENTED_EDGE ( 'NONE', *, *, #13967, .F. ) ;
#16209=CARTESIAN_POINT ( 'NONE',  ( 0.3042893218813439438, 6.450000000000000178, 2.170710678118660031 ) ) ;
#16246=FACE_OUTER_BOUND ( 'NONE', #4466, .T. ) ;
#16247=DIRECTION ( 'NONE',  ( 0.000000000000000000, 0.000000000000000000, 1.000000000000000000 ) ) ;
#16266=VERTEX_POINT ( 'NONE', #2844 ) ;
#16304=EDGE_LOOP ( 'NONE', ( #3234, #18058, #3374, #12771 ) ) ;
#16312=VERTEX_POINT ( 'NONE', #9695 ) ;
#16318=ORIENTED_EDGE ( 'NONE', *, *, #18174, .T. ) ;
#16352=VERTEX_POINT ( 'NONE', #10329 ) ;
#16354=DIRECTION ( 'NONE',  ( 1.224646799147350002E-16, -1.000000000000000000, -6.123233995736779594E-17 ) ) ;
#16361=DIRECTION ( 'NONE',  ( 0.000000000000000000, 0.000000000000000000, 1.000000000000000000 ) ) ;
#16398=LINE ( 'NONE', #9350, #3658 ) ;
#16449=DIRECTION ( 'NONE',  ( 1.224646799147350002E-16, -1.000000000000000000, -6.123233995736779594E-17 ) ) ;
#16493=VERTEX_POINT ( 'NONE', #17440 ) ;
#16498=ORIENTED_EDGE ( 'NONE', *, *, #10185, .T. ) ;
#16516=ADVANCED_FACE ( 'NONE', ( #16246 ), #12269, .T. ) ;
#16520=AXIS2_PLACEMENT_3D ( 'NONE', #14741, #17682, #668 ) ;
#16546=ORIENTED_EDGE ( 'NONE', *, *, #14331, .T. ) ;
#16558=CARTESIAN_POINT ( 'NONE',  ( 0.6207106781186539912, 6.450000000000000178, 2.628553390593269423 ) ) ;
#16562=EDGE_CURVE ( 'NONE', #9239, #2742, #7916, .T. ) ;
#16567=FACE_OUTER_BOUND ( 'NONE', #14511, .T. ) ;
#16571=EDGE_LOOP ( 'NONE', ( #6812, #4905, #15688, #11092 ) ) ;
#16575=ADVANCED_FACE ( 'NONE', ( #2075 ), #10881, .F. ) ;
#16628=ORIENTED_EDGE ( 'NONE', *, *, #14600, .F. ) ;
#16654=LINE ( 'NONE', #2113, #10647 ) ;
#16662=EDGE_CURVE ( 'NONE', #6139, #6673, #9070, .T. ) ;
#16678=DIRECTION ( 'NONE',  ( 1.000000000000000000, 0.000000000000000000, 0.000000000000000000 ) ) ;
#16698=ORIENTED_EDGE ( 'NONE', *, *, #9850, .T. ) ;
#16702=CARTESIAN_POINT ( 'NONE',  ( -0.6628679656440369383, 6.450000000000000178, 1.670710678118660031 ) ) ;
#16713=EDGE_CURVE ( 'NONE', #10138, #13931, #15340, .T. ) ;
#16717=CARTESIAN_POINT ( 'NONE',  ( 0.5500000000000000444, 6.450000000000000178, 3.200000000000000178 ) ) ;
#16724=VECTOR ( 'NONE', #13657, 1000.000000000000000 ) ;
#16738=FACE_OUTER_BOUND ( 'NONE', #11783, .T. ) ;
#16748=CARTESIAN_POINT ( 'NONE',  ( -0.6628679656440369383, 6.450000000000000178, 1.670710678118660031 ) ) ;
#16750=DIRECTION ( 'NONE',  ( -1.224646799147351975E-16, 1.000000000000000000, 6.123233995736759873E-17 ) ) ;
#16780=EDGE_LOOP ( 'NONE', ( #181, #1498, #11818, #8868 ) ) ;
#16787=CARTESIAN_POINT ( 'NONE',  ( -0.6914213562373099364, 6.450000000000000178, 2.557842712474620139 ) ) ;
#16793=ORIENTED_EDGE ( 'NONE', *, *, #11569, .F. ) ;
#16797=CIRCLE ( 'NONE', #8224, 0.2000000000000000389 ) ;
#16799=AXIS2_PLACEMENT_3D ( 'NONE', #10181, #6206, #5935 ) ;
#16803=AXIS2_PLACEMENT_3D ( 'NONE', #74, #16998, #4314 ) ;
#16818=VECTOR ( 'NONE', #7330, 1000.000000000000000 ) ;
#16824=VERTEX_POINT ( 'NONE', #12367 ) ;
#16833=ORIENTED_EDGE ( 'NONE', *, *, #9390, .F. ) ;
#16835=DIRECTION ( 'NONE',  ( 0.000000000000000000, -1.000000000000000000, 6.530723674265619530E-17 ) ) ;
#16836=DIRECTION ( 'NONE',  ( 0.000000000000000000, 0.000000000000000000, 1.000000000000000000 ) ) ;
#16841=DIRECTION ( 'NONE',  ( -2.612289469706250277E-16, 1.000000000000000000, 0.000000000000000000 ) ) ;
#16846=PLANE ( 'NONE',  #3737 ) ;
#16848=ADVANCED_FACE ( 'NONE', ( #8194 ), #14021, .T. ) ;
#16855=LINE ( 'NONE', #12788, #9765 ) ;
#16870=VECTOR ( 'NONE', #5967, 1000.000000000000000 ) ;
#16906=CARTESIAN_POINT ( 'NONE',  ( -0.6500000000000000222, 3.050000000000000266, 3.200000000000000178 ) ) ;
#16923=CARTESIAN_POINT ( 'NONE',  ( -0.6914213562373099364, 6.450000000000000178, 2.557842712474620139 ) ) ;
#16925=PLANE ( 'NONE',  #10007 ) ;
#16929=DIRECTION ( 'NONE',  ( 1.224646799147350002E-16, -1.000000000000000000, -6.123233995736769734E-17 ) ) ;
#16933=LINE ( 'NONE', #1922, #9334 ) ;
#16951=DIRECTION ( 'NONE',  ( -0.7071067811865489050, 0.000000000000000000, 0.7071067811865461294 ) ) ;
#16963=EDGE_CURVE ( 'NONE', #3787, #17050, #7468, .T. ) ;
#16983=ORIENTED_EDGE ( 'NONE', *, *, #15192, .T. ) ;
#16998=DIRECTION ( 'NONE',  ( 1.224646799147350002E-16, -1.000000000000000000, -6.123233995736769734E-17 ) ) ;
#17010=ORIENTED_EDGE ( 'NONE', *, *, #12357, .F. ) ;
#17020=ORIENTED_EDGE ( 'NONE', *, *, #12220, .F. ) ;
#17050=VERTEX_POINT ( 'NONE', #12273 ) ;
#17058=EDGE_CURVE ( 'NONE', #5909, #268, #15632, .T. ) ;
#17076=ORIENTED_EDGE ( 'NONE', *, *, #16662, .F. ) ;
#17093=ORIENTED_EDGE ( 'NONE', *, *, #11410, .T. ) ;
#17095=PLANE ( 'NONE',  #10359 ) ;
#17147=LINE ( 'NONE', #5697, #2861 ) ;
#17151=CARTESIAN_POINT ( 'NONE',  ( 0.5500000000000000444, 6.450000000000000178, 3.399999999999999911 ) ) ;
#17156=LINE ( 'NONE', #6052, #16870 ) ;
#17177=CARTESIAN_POINT ( 'NONE',  ( 0.2335786437626899970, 3.050000000000000266, 1.958578643762689753 ) ) ;
#17181=CARTESIAN_POINT ( 'NONE',  ( 0.6914213562373080491, 6.450000000000000178, 2.557842712474620139 ) ) ;
#17182=DIRECTION ( 'NONE',  ( 0.7071067811865480168, 0.000000000000000000, -0.7071067811865470176 ) ) ;
#17229=DIRECTION ( 'NONE',  ( 0.7071067811865474617, 0.000000000000000000, -0.7071067811865474617 ) ) ;
#17262=ORIENTED_EDGE ( 'NONE', *, *, #7123, .F. ) ;
#17266=DIRECTION ( 'NONE',  ( 1.224646799147350002E-16, -1.000000000000000000, -6.123233995736769734E-17 ) ) ;
#17288=SURFACE_STYLE_FILL_AREA ( #17394 ) ;
#17382=LINE ( 'NONE', #7407, #1483 ) ;
#17386=LINE ( 'NONE', #4989, #2601 ) ;
#17394=FILL_AREA_STYLE ('',( #11766 ) ) ;
#17414=PRODUCT_DEFINITION_FORMATION_WITH_SPECIFIED_SOURCE ( 'ANY', '', #8021, .NOT_KNOWN. ) ;
#17425=CARTESIAN_POINT ( 'NONE',  ( -0.3042893218813459977, 6.450000000000000178, 2.170710678118660031 ) ) ;
#17440=CARTESIAN_POINT ( 'NONE',  ( -0.5921572875253809931, 3.050000000000000266, 1.600000000000000089 ) ) ;
#17456=VECTOR ( 'NONE', #16124, 1000.000000000000000 ) ;
#17493=EDGE_CURVE ( 'NONE', #9105, #16183, #16797, .T. ) ;
#17528=DIRECTION ( 'NONE',  ( -1.000000000000000000, 0.000000000000000000, 0.000000000000000000 ) ) ;
#17568=EDGE_LOOP ( 'NONE', ( #10677, #8399, #12990, #6028 ) ) ;
#17618=ORIENTED_EDGE ( 'NONE', *, *, #12249, .F. ) ;
#17619=CARTESIAN_POINT ( 'NONE',  ( 0.6500000000000000222, 6.450000000000000178, 3.200000000000000178 ) ) ;
#17652=VERTEX_POINT ( 'NONE', #16906 ) ;
#17681=AXIS2_PLACEMENT_3D ( 'NONE', #11191, #16836, #4146 ) ;
#17682=DIRECTION ( 'NONE',  ( 1.224646799147351975E-16, -1.000000000000000000, -6.123233995736789455E-17 ) ) ;
#17707=DIRECTION ( 'NONE',  ( -1.224646799147350002E-16, 1.000000000000000000, 6.123233995736769734E-17 ) ) ;
#17726=EDGE_CURVE ( 'NONE', #3220, #10706, #7627, .T. ) ;
#17797=DIRECTION ( 'NONE',  ( 0.7071067811865470176, 0.000000000000000000, -0.7071067811865480168 ) ) ;
#17811=CARTESIAN_POINT ( 'NONE',  ( 0.3750000000000000000, 3.050000000000000266, 2.100000000000000089 ) ) ;
#17840=CARTESIAN_POINT ( 'NONE',  ( -0.3042893218813459977, 6.450000000000000178, 2.029289321881350361 ) ) ;
#17859=PRODUCT_DEFINITION_CONTEXT ( 'detailed design', #2003, 'design' ) ;
#17860=VERTEX_POINT ( 'NONE', #15325 ) ;
#17861=DIRECTION ( 'NONE',  ( 1.224646799147350002E-16, -1.000000000000000000, -6.123233995736769734E-17 ) ) ;
#17864=LINE ( 'NONE', #1043, #9424 ) ;
#17900=LINE ( 'NONE', #13673, #1200 ) ;
#17924=DIRECTION ( 'NONE',  ( -0.7071067811865474617, 0.000000000000000000, -0.7071067811865474617 ) ) ;
#17947=EDGE_CURVE ( 'NONE', #8985, #8650, #12444, .T. ) ;
#17958=CARTESIAN_POINT ( 'NONE',  ( -0.6500000000000000222, 6.450000000000000178, 2.699264068711930253 ) ) ;
#18040=ORIENTED_EDGE ( 'NONE', *, *, #15933, .T. ) ;
#18058=ORIENTED_EDGE ( 'NONE', *, *, #12813, .T. ) ;
#18061=ORIENTED_EDGE ( 'NONE', *, *, #12779, .F. ) ;
#18073=DIRECTION ( 'NONE',  ( 0.000000000000000000, 0.000000000000000000, 1.000000000000000000 ) ) ;
#18085=DIRECTION ( 'NONE',  ( -1.306144734853129823E-16, 1.000000000000000000, 0.000000000000000000 ) ) ;
#18096=EDGE_CURVE ( 'NONE', #10706, #5909, #6383, .T. ) ;
#18106=DIRECTION ( 'NONE',  ( 0.7071067811865475727, 4.617918996128745560E-17, 0.7071067811865475727 ) ) ;
#18109=ORIENTED_EDGE ( 'NONE', *, *, #1896, .T. ) ;
#18122=ORIENTED_EDGE ( 'NONE', *, *, #15801, .F. ) ;
#18140=DIRECTION ( 'NONE',  ( 9.796085511398438540E-17, -1.000000000000000000, 0.000000000000000000 ) ) ;
#18141=ORIENTED_EDGE ( 'NONE', *, *, #17493, .T. ) ;
#18174=EDGE_CURVE ( 'NONE', #12759, #7292, #2009, .T. ) ;
#18217=ORIENTED_EDGE ( 'NONE', *, *, #7463, .T. ) ;
#18231=VECTOR ( 'NONE', #7994, 1000.000000000000000 ) ;
#18236=LINE ( 'NONE', #9844, #14483 ) ;
#18247=AXIS2_PLACEMENT_3D ( 'NONE', #17840, #9537, #16841 ) ;
#18272=ORIENTED_EDGE ( 'NONE', *, *, #14600, .T. ) ;
ENDSEC;
END-ISO-10303-21;
